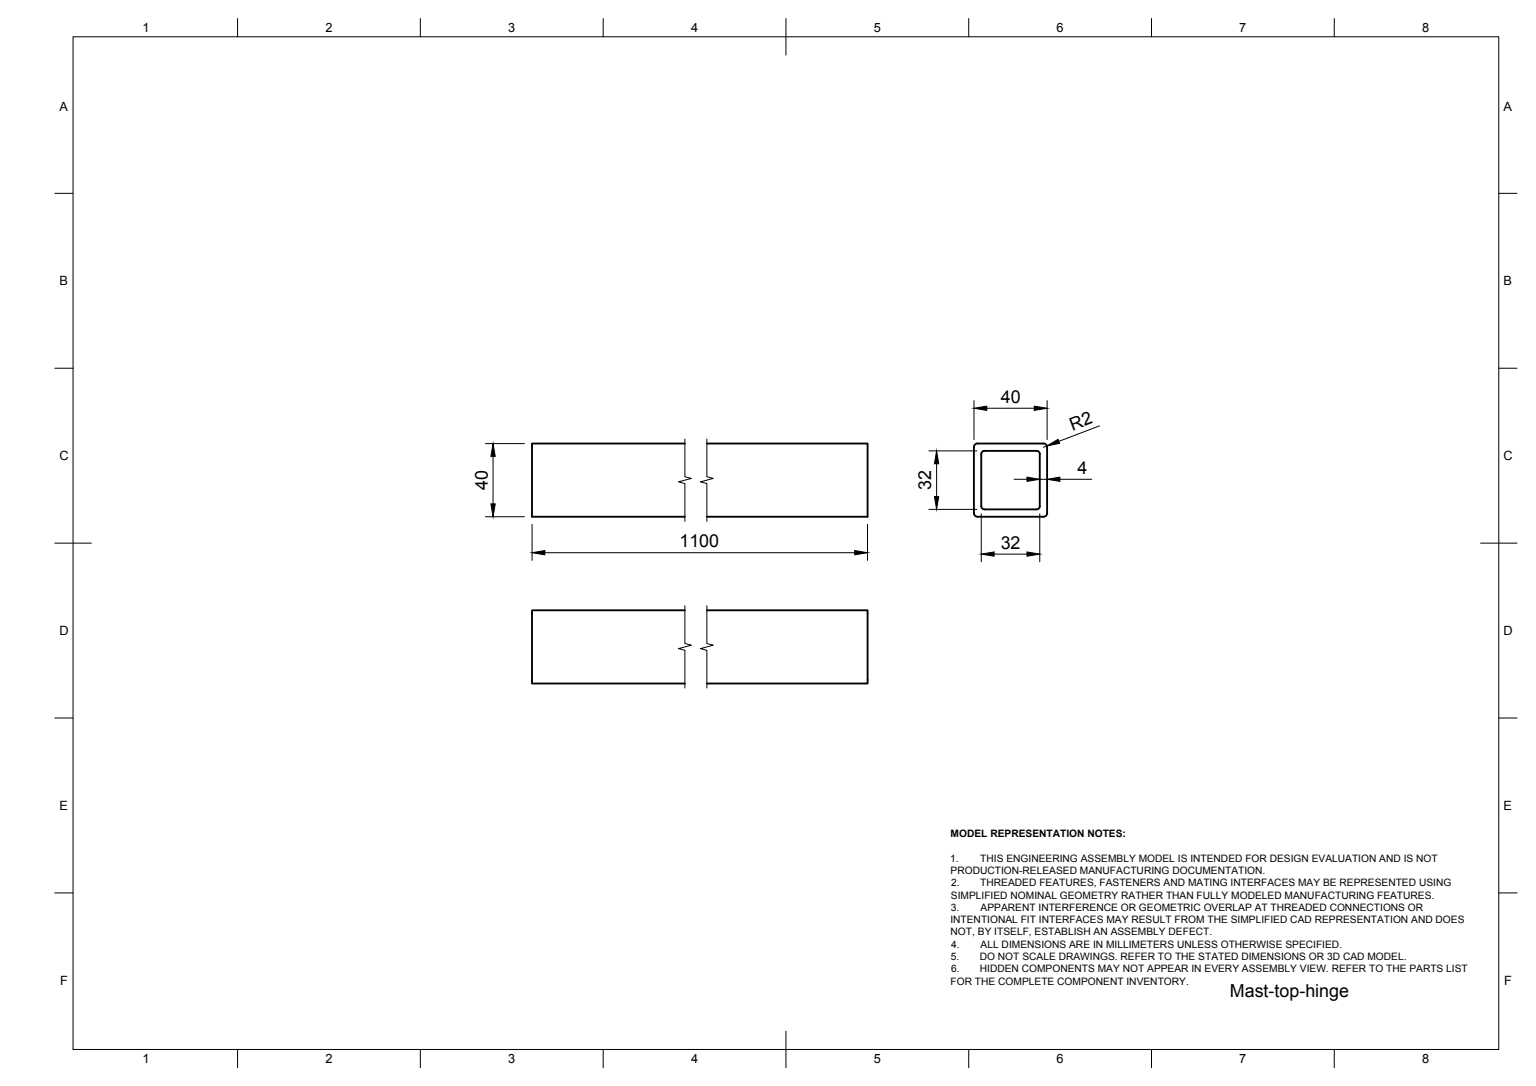
ISO-10303-21;
HEADER;
/* Generated by software containing ST-Developer
 * from STEP Tools, Inc. (www.steptools.com) 
 */

FILE_DESCRIPTION(
/* description */ (''),
/* implementation_level */ '2;1');

FILE_NAME(
/* name */ 'Mast-top-hinge.step',
/* time_stamp */ '2026-10-07T11:02:43-07:00',
/* author */ (''),
/* organization */ (''),
/* preprocessor_version */ 'ST-DEVELOPER v20.2',
/* originating_system */ 'Autodesk Translation Framework v15.15.0.0',
/* authorisation */ '');

FILE_SCHEMA (('AUTOMOTIVE_DESIGN { 1 0 10303 214 3 1 1 }'));
ENDSEC;

DATA;
#10=MECHANICAL_DESIGN_GEOMETRIC_PRESENTATION_REPRESENTATION('',(#67),#5505);
#53=SHAPE_REPRESENTATION_RELATIONSHIP('SRR','None',#5538,#60);
#60=ADVANCED_BREP_SHAPE_REPRESENTATION('',(#74),#5499);
#67=STYLED_ITEM('',(#5582),#74);
#74=MANIFOLD_SOLID_BREP('Body1',#3294);
#84=FACE_BOUND('',#447,.T.);
#85=FACE_BOUND('',#448,.T.);
#86=FACE_BOUND('',#450,.T.);
#87=FACE_BOUND('',#451,.T.);
#88=FACE_BOUND('',#461,.T.);
#89=FACE_BOUND('',#462,.T.);
#90=FACE_BOUND('',#463,.T.);
#91=FACE_BOUND('',#464,.T.);
#92=FACE_BOUND('',#466,.T.);
#93=FACE_BOUND('',#467,.T.);
#94=FACE_BOUND('',#468,.T.);
#95=FACE_BOUND('',#469,.T.);
#96=FACE_BOUND('',#477,.T.);
#97=FACE_BOUND('',#479,.T.);
#121=CYLINDRICAL_SURFACE('',#3450,2.);
#122=CYLINDRICAL_SURFACE('',#3453,2.);
#123=CYLINDRICAL_SURFACE('',#3457,2.);
#124=CYLINDRICAL_SURFACE('',#3460,2.);
#125=CYLINDRICAL_SURFACE('',#3473,1.8);
#126=CYLINDRICAL_SURFACE('',#3474,1.8);
#127=CYLINDRICAL_SURFACE('',#3476,1.8);
#128=CYLINDRICAL_SURFACE('',#3477,1.8);
#169=CIRCLE('',#3451,2.);
#170=CIRCLE('',#3452,2.);
#171=CIRCLE('',#3454,2.);
#172=CIRCLE('',#3455,2.);
#173=CIRCLE('',#3458,2.);
#174=CIRCLE('',#3459,2.);
#175=CIRCLE('',#3461,2.);
#176=CIRCLE('',#3462,2.);
#177=CIRCLE('',#3464,1.8);
#178=CIRCLE('',#3465,1.8);
#179=CIRCLE('',#3466,1.8);
#180=CIRCLE('',#3467,1.8);
#181=CIRCLE('',#3469,1.8);
#182=CIRCLE('',#3470,1.8);
#183=CIRCLE('',#3471,1.8);
#184=CIRCLE('',#3472,1.8);
#276=FACE_OUTER_BOUND('',#446,.T.);
#277=FACE_OUTER_BOUND('',#449,.T.);
#278=FACE_OUTER_BOUND('',#452,.T.);
#279=FACE_OUTER_BOUND('',#453,.T.);
#280=FACE_OUTER_BOUND('',#454,.T.);
#281=FACE_OUTER_BOUND('',#455,.T.);
#282=FACE_OUTER_BOUND('',#456,.T.);
#283=FACE_OUTER_BOUND('',#457,.T.);
#284=FACE_OUTER_BOUND('',#458,.T.);
#285=FACE_OUTER_BOUND('',#459,.T.);
#286=FACE_OUTER_BOUND('',#460,.T.);
#287=FACE_OUTER_BOUND('',#465,.T.);
#288=FACE_OUTER_BOUND('',#470,.T.);
#289=FACE_OUTER_BOUND('',#471,.T.);
#290=FACE_OUTER_BOUND('',#472,.T.);
#291=FACE_OUTER_BOUND('',#473,.T.);
#292=FACE_OUTER_BOUND('',#474,.T.);
#293=FACE_OUTER_BOUND('',#475,.T.);
#294=FACE_OUTER_BOUND('',#476,.T.);
#295=FACE_OUTER_BOUND('',#478,.T.);
#296=FACE_OUTER_BOUND('',#480,.T.);
#297=FACE_OUTER_BOUND('',#481,.T.);
#298=FACE_OUTER_BOUND('',#482,.T.);
#299=FACE_OUTER_BOUND('',#483,.T.);
#300=FACE_OUTER_BOUND('',#484,.T.);
#301=FACE_OUTER_BOUND('',#485,.T.);
#302=FACE_OUTER_BOUND('',#486,.T.);
#303=FACE_OUTER_BOUND('',#487,.T.);
#304=FACE_OUTER_BOUND('',#488,.T.);
#305=FACE_OUTER_BOUND('',#489,.T.);
#306=FACE_OUTER_BOUND('',#490,.T.);
#307=FACE_OUTER_BOUND('',#491,.T.);
#308=FACE_OUTER_BOUND('',#492,.T.);
#309=FACE_OUTER_BOUND('',#493,.T.);
#310=FACE_OUTER_BOUND('',#494,.T.);
#311=FACE_OUTER_BOUND('',#495,.T.);
#312=FACE_OUTER_BOUND('',#496,.T.);
#313=FACE_OUTER_BOUND('',#497,.T.);
#314=FACE_OUTER_BOUND('',#498,.T.);
#315=FACE_OUTER_BOUND('',#499,.T.);
#316=FACE_OUTER_BOUND('',#500,.T.);
#317=FACE_OUTER_BOUND('',#501,.T.);
#446=EDGE_LOOP('',(#2336,#2337,#2338,#2339));
#447=EDGE_LOOP('',(#2340,#2341,#2342,#2343));
#448=EDGE_LOOP('',(#2344,#2345,#2346,#2347));
#449=EDGE_LOOP('',(#2348,#2349,#2350,#2351));
#450=EDGE_LOOP('',(#2352,#2353,#2354,#2355));
#451=EDGE_LOOP('',(#2356,#2357,#2358,#2359));
#452=EDGE_LOOP('',(#2360,#2361,#2362,#2363));
#453=EDGE_LOOP('',(#2364,#2365,#2366,#2367));
#454=EDGE_LOOP('',(#2368,#2369,#2370,#2371));
#455=EDGE_LOOP('',(#2372,#2373,#2374,#2375));
#456=EDGE_LOOP('',(#2376,#2377,#2378,#2379));
#457=EDGE_LOOP('',(#2380,#2381,#2382,#2383));
#458=EDGE_LOOP('',(#2384,#2385,#2386,#2387));
#459=EDGE_LOOP('',(#2388,#2389,#2390,#2391));
#460=EDGE_LOOP('',(#2392,#2393,#2394,#2395));
#461=EDGE_LOOP('',(#2396,#2397,#2398,#2399));
#462=EDGE_LOOP('',(#2400,#2401,#2402,#2403));
#463=EDGE_LOOP('',(#2404,#2405,#2406,#2407));
#464=EDGE_LOOP('',(#2408,#2409,#2410,#2411));
#465=EDGE_LOOP('',(#2412,#2413,#2414,#2415));
#466=EDGE_LOOP('',(#2416,#2417,#2418,#2419));
#467=EDGE_LOOP('',(#2420,#2421,#2422,#2423));
#468=EDGE_LOOP('',(#2424,#2425,#2426,#2427));
#469=EDGE_LOOP('',(#2428,#2429,#2430,#2431));
#470=EDGE_LOOP('',(#2432,#2433,#2434,#2435));
#471=EDGE_LOOP('',(#2436,#2437,#2438,#2439));
#472=EDGE_LOOP('',(#2440,#2441,#2442,#2443));
#473=EDGE_LOOP('',(#2444,#2445,#2446,#2447));
#474=EDGE_LOOP('',(#2448,#2449,#2450,#2451));
#475=EDGE_LOOP('',(#2452,#2453,#2454,#2455));
#476=EDGE_LOOP('',(#2456,#2457,#2458,#2459,#2460,#2461,#2462,#2463));
#477=EDGE_LOOP('',(#2464,#2465,#2466,#2467,#2468,#2469,#2470,#2471));
#478=EDGE_LOOP('',(#2472,#2473,#2474,#2475,#2476,#2477,#2478,#2479));
#479=EDGE_LOOP('',(#2480,#2481,#2482,#2483,#2484,#2485,#2486,#2487));
#480=EDGE_LOOP('',(#2488,#2489,#2490,#2491));
#481=EDGE_LOOP('',(#2492,#2493,#2494,#2495));
#482=EDGE_LOOP('',(#2496,#2497,#2498,#2499));
#483=EDGE_LOOP('',(#2500,#2501,#2502,#2503));
#484=EDGE_LOOP('',(#2504,#2505,#2506,#2507));
#485=EDGE_LOOP('',(#2508,#2509,#2510,#2511));
#486=EDGE_LOOP('',(#2512,#2513,#2514,#2515));
#487=EDGE_LOOP('',(#2516,#2517,#2518,#2519));
#488=EDGE_LOOP('',(#2520,#2521,#2522,#2523));
#489=EDGE_LOOP('',(#2524,#2525,#2526,#2527));
#490=EDGE_LOOP('',(#2528,#2529,#2530,#2531));
#491=EDGE_LOOP('',(#2532,#2533,#2534,#2535));
#492=EDGE_LOOP('',(#2536,#2537,#2538,#2539));
#493=EDGE_LOOP('',(#2540,#2541,#2542,#2543));
#494=EDGE_LOOP('',(#2544,#2545,#2546,#2547));
#495=EDGE_LOOP('',(#2548,#2549,#2550,#2551));
#496=EDGE_LOOP('',(#2552,#2553,#2554,#2555));
#497=EDGE_LOOP('',(#2556,#2557,#2558,#2559));
#498=EDGE_LOOP('',(#2560,#2561,#2562,#2563));
#499=EDGE_LOOP('',(#2564,#2565,#2566,#2567));
#500=EDGE_LOOP('',(#2568,#2569,#2570,#2571));
#501=EDGE_LOOP('',(#2572,#2573,#2574,#2575));
#705=LINE('',#4795,#1075);
#706=LINE('',#4797,#1076);
#707=LINE('',#4799,#1077);
#708=LINE('',#4800,#1078);
#709=LINE('',#4803,#1079);
#710=LINE('',#4805,#1080);
#711=LINE('',#4807,#1081);
#712=LINE('',#4808,#1082);
#713=LINE('',#4811,#1083);
#714=LINE('',#4813,#1084);
#715=LINE('',#4815,#1085);
#716=LINE('',#4816,#1086);
#717=LINE('',#4820,#1087);
#718=LINE('',#4822,#1088);
#719=LINE('',#4824,#1089);
#720=LINE('',#4825,#1090);
#721=LINE('',#4828,#1091);
#722=LINE('',#4830,#1092);
#723=LINE('',#4832,#1093);
#724=LINE('',#4833,#1094);
#725=LINE('',#4836,#1095);
#726=LINE('',#4838,#1096);
#727=LINE('',#4840,#1097);
#728=LINE('',#4841,#1098);
#729=LINE('',#4845,#1099);
#730=LINE('',#4847,#1100);
#731=LINE('',#4849,#1101);
#732=LINE('',#4850,#1102);
#733=LINE('',#4853,#1103);
#734=LINE('',#4855,#1104);
#735=LINE('',#4856,#1105);
#736=LINE('',#4859,#1106);
#737=LINE('',#4861,#1107);
#738=LINE('',#4862,#1108);
#739=LINE('',#4864,#1109);
#740=LINE('',#4865,#1110);
#741=LINE('',#4869,#1111);
#742=LINE('',#4871,#1112);
#743=LINE('',#4873,#1113);
#744=LINE('',#4874,#1114);
#745=LINE('',#4877,#1115);
#746=LINE('',#4879,#1116);
#747=LINE('',#4880,#1117);
#748=LINE('',#4883,#1118);
#749=LINE('',#4885,#1119);
#750=LINE('',#4886,#1120);
#751=LINE('',#4888,#1121);
#752=LINE('',#4889,#1122);
#753=LINE('',#4893,#1123);
#754=LINE('',#4895,#1124);
#755=LINE('',#4897,#1125);
#756=LINE('',#4898,#1126);
#757=LINE('',#4901,#1127);
#758=LINE('',#4903,#1128);
#759=LINE('',#4905,#1129);
#760=LINE('',#4906,#1130);
#761=LINE('',#4909,#1131);
#762=LINE('',#4911,#1132);
#763=LINE('',#4913,#1133);
#764=LINE('',#4914,#1134);
#765=LINE('',#4918,#1135);
#766=LINE('',#4920,#1136);
#767=LINE('',#4922,#1137);
#768=LINE('',#4923,#1138);
#769=LINE('',#4926,#1139);
#770=LINE('',#4928,#1140);
#771=LINE('',#4930,#1141);
#772=LINE('',#4931,#1142);
#773=LINE('',#4934,#1143);
#774=LINE('',#4936,#1144);
#775=LINE('',#4938,#1145);
#776=LINE('',#4939,#1146);
#777=LINE('',#4943,#1147);
#778=LINE('',#4945,#1148);
#779=LINE('',#4947,#1149);
#780=LINE('',#4948,#1150);
#781=LINE('',#4956,#1151);
#782=LINE('',#4960,#1152);
#783=LINE('',#4962,#1153);
#784=LINE('',#4963,#1154);
#785=LINE('',#4976,#1155);
#786=LINE('',#4980,#1156);
#787=LINE('',#4985,#1157);
#788=LINE('',#4990,#1158);
#789=LINE('',#4993,#1159);
#790=LINE('',#4995,#1160);
#791=LINE('',#4997,#1161);
#792=LINE('',#5000,#1162);
#793=LINE('',#5003,#1163);
#794=LINE('',#5004,#1164);
#795=LINE('',#5006,#1165);
#796=LINE('',#5008,#1166);
#797=LINE('',#5011,#1167);
#798=LINE('',#5012,#1168);
#799=LINE('',#5014,#1169);
#800=LINE('',#5016,#1170);
#801=LINE('',#5019,#1171);
#802=LINE('',#5020,#1172);
#803=LINE('',#5022,#1173);
#804=LINE('',#5024,#1174);
#805=LINE('',#5027,#1175);
#806=LINE('',#5028,#1176);
#807=LINE('',#5030,#1177);
#808=LINE('',#5032,#1178);
#1075=VECTOR('',#3869,1000.);
#1076=VECTOR('',#3870,1000.);
#1077=VECTOR('',#3871,1000.);
#1078=VECTOR('',#3872,1000.);
#1079=VECTOR('',#3873,1000.);
#1080=VECTOR('',#3874,1000.);
#1081=VECTOR('',#3875,1000.);
#1082=VECTOR('',#3876,1000.);
#1083=VECTOR('',#3877,1000.);
#1084=VECTOR('',#3878,1000.);
#1085=VECTOR('',#3879,1000.);
#1086=VECTOR('',#3880,1000.);
#1087=VECTOR('',#3883,1000.);
#1088=VECTOR('',#3884,1000.);
#1089=VECTOR('',#3885,1000.);
#1090=VECTOR('',#3886,1000.);
#1091=VECTOR('',#3887,1000.);
#1092=VECTOR('',#3888,1000.);
#1093=VECTOR('',#3889,1000.);
#1094=VECTOR('',#3890,1000.);
#1095=VECTOR('',#3891,1000.);
#1096=VECTOR('',#3892,1000.);
#1097=VECTOR('',#3893,1000.);
#1098=VECTOR('',#3894,1000.);
#1099=VECTOR('',#3897,1000.);
#1100=VECTOR('',#3898,1000.);
#1101=VECTOR('',#3899,1000.);
#1102=VECTOR('',#3900,1000.);
#1103=VECTOR('',#3903,1000.);
#1104=VECTOR('',#3904,1000.);
#1105=VECTOR('',#3905,1000.);
#1106=VECTOR('',#3908,1000.);
#1107=VECTOR('',#3909,1000.);
#1108=VECTOR('',#3910,1000.);
#1109=VECTOR('',#3913,1000.);
#1110=VECTOR('',#3914,1000.);
#1111=VECTOR('',#3917,1000.);
#1112=VECTOR('',#3918,1000.);
#1113=VECTOR('',#3919,1000.);
#1114=VECTOR('',#3920,1000.);
#1115=VECTOR('',#3923,1000.);
#1116=VECTOR('',#3924,1000.);
#1117=VECTOR('',#3925,1000.);
#1118=VECTOR('',#3928,1000.);
#1119=VECTOR('',#3929,1000.);
#1120=VECTOR('',#3930,1000.);
#1121=VECTOR('',#3933,1000.);
#1122=VECTOR('',#3934,1000.);
#1123=VECTOR('',#3937,1000.);
#1124=VECTOR('',#3938,1000.);
#1125=VECTOR('',#3939,1000.);
#1126=VECTOR('',#3940,1000.);
#1127=VECTOR('',#3941,1000.);
#1128=VECTOR('',#3942,1000.);
#1129=VECTOR('',#3943,1000.);
#1130=VECTOR('',#3944,1000.);
#1131=VECTOR('',#3945,1000.);
#1132=VECTOR('',#3946,1000.);
#1133=VECTOR('',#3947,1000.);
#1134=VECTOR('',#3948,1000.);
#1135=VECTOR('',#3951,1000.);
#1136=VECTOR('',#3952,1000.);
#1137=VECTOR('',#3953,1000.);
#1138=VECTOR('',#3954,1000.);
#1139=VECTOR('',#3955,1000.);
#1140=VECTOR('',#3956,1000.);
#1141=VECTOR('',#3957,1000.);
#1142=VECTOR('',#3958,1000.);
#1143=VECTOR('',#3959,1000.);
#1144=VECTOR('',#3960,1000.);
#1145=VECTOR('',#3961,1000.);
#1146=VECTOR('',#3962,1000.);
#1147=VECTOR('',#3965,1000.);
#1148=VECTOR('',#3966,1000.);
#1149=VECTOR('',#3967,1000.);
#1150=VECTOR('',#3968,1000.);
#1151=VECTOR('',#3979,1000.);
#1152=VECTOR('',#3984,1000.);
#1153=VECTOR('',#3985,1000.);
#1154=VECTOR('',#3986,1000.);
#1155=VECTOR('',#4005,1000.);
#1156=VECTOR('',#4010,1000.);
#1157=VECTOR('',#4015,1000.);
#1158=VECTOR('',#4020,1000.);
#1159=VECTOR('',#4025,1000.);
#1160=VECTOR('',#4028,1000.);
#1161=VECTOR('',#4031,1000.);
#1162=VECTOR('',#4036,1000.);
#1163=VECTOR('',#4041,1000.);
#1164=VECTOR('',#4042,1000.);
#1165=VECTOR('',#4045,1000.);
#1166=VECTOR('',#4048,1000.);
#1167=VECTOR('',#4053,1000.);
#1168=VECTOR('',#4054,1000.);
#1169=VECTOR('',#4057,1000.);
#1170=VECTOR('',#4060,1000.);
#1171=VECTOR('',#4065,1000.);
#1172=VECTOR('',#4066,1000.);
#1173=VECTOR('',#4069,1000.);
#1174=VECTOR('',#4072,1000.);
#1175=VECTOR('',#4077,1000.);
#1176=VECTOR('',#4078,1000.);
#1177=VECTOR('',#4081,1000.);
#1178=VECTOR('',#4084,1000.);
#1421=VERTEX_POINT('',#4793);
#1422=VERTEX_POINT('',#4794);
#1423=VERTEX_POINT('',#4796);
#1424=VERTEX_POINT('',#4798);
#1425=VERTEX_POINT('',#4801);
#1426=VERTEX_POINT('',#4802);
#1427=VERTEX_POINT('',#4804);
#1428=VERTEX_POINT('',#4806);
#1429=VERTEX_POINT('',#4809);
#1430=VERTEX_POINT('',#4810);
#1431=VERTEX_POINT('',#4812);
#1432=VERTEX_POINT('',#4814);
#1433=VERTEX_POINT('',#4818);
#1434=VERTEX_POINT('',#4819);
#1435=VERTEX_POINT('',#4821);
#1436=VERTEX_POINT('',#4823);
#1437=VERTEX_POINT('',#4826);
#1438=VERTEX_POINT('',#4827);
#1439=VERTEX_POINT('',#4829);
#1440=VERTEX_POINT('',#4831);
#1441=VERTEX_POINT('',#4834);
#1442=VERTEX_POINT('',#4835);
#1443=VERTEX_POINT('',#4837);
#1444=VERTEX_POINT('',#4839);
#1445=VERTEX_POINT('',#4843);
#1446=VERTEX_POINT('',#4844);
#1447=VERTEX_POINT('',#4846);
#1448=VERTEX_POINT('',#4848);
#1449=VERTEX_POINT('',#4852);
#1450=VERTEX_POINT('',#4854);
#1451=VERTEX_POINT('',#4858);
#1452=VERTEX_POINT('',#4860);
#1453=VERTEX_POINT('',#4867);
#1454=VERTEX_POINT('',#4868);
#1455=VERTEX_POINT('',#4870);
#1456=VERTEX_POINT('',#4872);
#1457=VERTEX_POINT('',#4876);
#1458=VERTEX_POINT('',#4878);
#1459=VERTEX_POINT('',#4882);
#1460=VERTEX_POINT('',#4884);
#1461=VERTEX_POINT('',#4891);
#1462=VERTEX_POINT('',#4892);
#1463=VERTEX_POINT('',#4894);
#1464=VERTEX_POINT('',#4896);
#1465=VERTEX_POINT('',#4899);
#1466=VERTEX_POINT('',#4900);
#1467=VERTEX_POINT('',#4902);
#1468=VERTEX_POINT('',#4904);
#1469=VERTEX_POINT('',#4907);
#1470=VERTEX_POINT('',#4908);
#1471=VERTEX_POINT('',#4910);
#1472=VERTEX_POINT('',#4912);
#1473=VERTEX_POINT('',#4916);
#1474=VERTEX_POINT('',#4917);
#1475=VERTEX_POINT('',#4919);
#1476=VERTEX_POINT('',#4921);
#1477=VERTEX_POINT('',#4924);
#1478=VERTEX_POINT('',#4925);
#1479=VERTEX_POINT('',#4927);
#1480=VERTEX_POINT('',#4929);
#1481=VERTEX_POINT('',#4932);
#1482=VERTEX_POINT('',#4933);
#1483=VERTEX_POINT('',#4935);
#1484=VERTEX_POINT('',#4937);
#1485=VERTEX_POINT('',#4941);
#1486=VERTEX_POINT('',#4942);
#1487=VERTEX_POINT('',#4944);
#1488=VERTEX_POINT('',#4946);
#1489=VERTEX_POINT('',#4953);
#1490=VERTEX_POINT('',#4955);
#1491=VERTEX_POINT('',#4959);
#1492=VERTEX_POINT('',#4961);
#1493=VERTEX_POINT('',#4971);
#1494=VERTEX_POINT('',#4973);
#1495=VERTEX_POINT('',#4975);
#1496=VERTEX_POINT('',#4978);
#1497=VERTEX_POINT('',#4982);
#1498=VERTEX_POINT('',#4984);
#1499=VERTEX_POINT('',#4987);
#1500=VERTEX_POINT('',#4989);
#1763=EDGE_CURVE('',#1421,#1422,#705,.T.);
#1764=EDGE_CURVE('',#1422,#1423,#706,.T.);
#1765=EDGE_CURVE('',#1424,#1423,#707,.T.);
#1766=EDGE_CURVE('',#1421,#1424,#708,.T.);
#1767=EDGE_CURVE('',#1425,#1426,#709,.T.);
#1768=EDGE_CURVE('',#1425,#1427,#710,.T.);
#1769=EDGE_CURVE('',#1427,#1428,#711,.T.);
#1770=EDGE_CURVE('',#1426,#1428,#712,.T.);
#1771=EDGE_CURVE('',#1429,#1430,#713,.T.);
#1772=EDGE_CURVE('',#1430,#1431,#714,.T.);
#1773=EDGE_CURVE('',#1432,#1431,#715,.T.);
#1774=EDGE_CURVE('',#1429,#1432,#716,.T.);
#1775=EDGE_CURVE('',#1433,#1434,#717,.T.);
#1776=EDGE_CURVE('',#1435,#1434,#718,.T.);
#1777=EDGE_CURVE('',#1436,#1435,#719,.T.);
#1778=EDGE_CURVE('',#1436,#1433,#720,.T.);
#1779=EDGE_CURVE('',#1437,#1438,#721,.T.);
#1780=EDGE_CURVE('',#1438,#1439,#722,.T.);
#1781=EDGE_CURVE('',#1440,#1439,#723,.T.);
#1782=EDGE_CURVE('',#1437,#1440,#724,.T.);
#1783=EDGE_CURVE('',#1441,#1442,#725,.T.);
#1784=EDGE_CURVE('',#1441,#1443,#726,.T.);
#1785=EDGE_CURVE('',#1443,#1444,#727,.T.);
#1786=EDGE_CURVE('',#1442,#1444,#728,.T.);
#1787=EDGE_CURVE('',#1445,#1446,#729,.T.);
#1788=EDGE_CURVE('',#1445,#1447,#730,.T.);
#1789=EDGE_CURVE('',#1447,#1448,#731,.T.);
#1790=EDGE_CURVE('',#1448,#1446,#732,.T.);
#1791=EDGE_CURVE('',#1447,#1449,#733,.T.);
#1792=EDGE_CURVE('',#1449,#1450,#734,.T.);
#1793=EDGE_CURVE('',#1450,#1448,#735,.T.);
#1794=EDGE_CURVE('',#1449,#1451,#736,.T.);
#1795=EDGE_CURVE('',#1451,#1452,#737,.T.);
#1796=EDGE_CURVE('',#1452,#1450,#738,.T.);
#1797=EDGE_CURVE('',#1451,#1445,#739,.T.);
#1798=EDGE_CURVE('',#1446,#1452,#740,.T.);
#1799=EDGE_CURVE('',#1453,#1454,#741,.T.);
#1800=EDGE_CURVE('',#1453,#1455,#742,.T.);
#1801=EDGE_CURVE('',#1455,#1456,#743,.T.);
#1802=EDGE_CURVE('',#1456,#1454,#744,.T.);
#1803=EDGE_CURVE('',#1457,#1455,#745,.T.);
#1804=EDGE_CURVE('',#1457,#1458,#746,.T.);
#1805=EDGE_CURVE('',#1456,#1458,#747,.T.);
#1806=EDGE_CURVE('',#1459,#1457,#748,.T.);
#1807=EDGE_CURVE('',#1459,#1460,#749,.T.);
#1808=EDGE_CURVE('',#1458,#1460,#750,.T.);
#1809=EDGE_CURVE('',#1459,#1453,#751,.T.);
#1810=EDGE_CURVE('',#1454,#1460,#752,.T.);
#1811=EDGE_CURVE('',#1461,#1462,#753,.T.);
#1812=EDGE_CURVE('',#1463,#1462,#754,.T.);
#1813=EDGE_CURVE('',#1464,#1463,#755,.T.);
#1814=EDGE_CURVE('',#1464,#1461,#756,.T.);
#1815=EDGE_CURVE('',#1465,#1466,#757,.T.);
#1816=EDGE_CURVE('',#1466,#1467,#758,.T.);
#1817=EDGE_CURVE('',#1467,#1468,#759,.T.);
#1818=EDGE_CURVE('',#1468,#1465,#760,.T.);
#1819=EDGE_CURVE('',#1469,#1470,#761,.T.);
#1820=EDGE_CURVE('',#1469,#1471,#762,.T.);
#1821=EDGE_CURVE('',#1471,#1472,#763,.T.);
#1822=EDGE_CURVE('',#1470,#1472,#764,.T.);
#1823=EDGE_CURVE('',#1473,#1474,#765,.T.);
#1824=EDGE_CURVE('',#1475,#1474,#766,.F.);
#1825=EDGE_CURVE('',#1476,#1475,#767,.T.);
#1826=EDGE_CURVE('',#1476,#1473,#768,.F.);
#1827=EDGE_CURVE('',#1477,#1478,#769,.T.);
#1828=EDGE_CURVE('',#1478,#1479,#770,.T.);
#1829=EDGE_CURVE('',#1479,#1480,#771,.T.);
#1830=EDGE_CURVE('',#1480,#1477,#772,.T.);
#1831=EDGE_CURVE('',#1481,#1482,#773,.T.);
#1832=EDGE_CURVE('',#1482,#1483,#774,.T.);
#1833=EDGE_CURVE('',#1484,#1483,#775,.T.);
#1834=EDGE_CURVE('',#1481,#1484,#776,.T.);
#1835=EDGE_CURVE('',#1485,#1486,#777,.T.);
#1836=EDGE_CURVE('',#1487,#1485,#778,.T.);
#1837=EDGE_CURVE('',#1487,#1488,#779,.T.);
#1838=EDGE_CURVE('',#1488,#1486,#780,.T.);
#1839=EDGE_CURVE('',#1474,#1485,#169,.T.);
#1840=EDGE_CURVE('',#1473,#1487,#170,.T.);
#1841=EDGE_CURVE('',#1489,#1475,#171,.T.);
#1842=EDGE_CURVE('',#1490,#1489,#781,.T.);
#1843=EDGE_CURVE('',#1490,#1476,#172,.T.);
#1844=EDGE_CURVE('',#1491,#1489,#782,.F.);
#1845=EDGE_CURVE('',#1492,#1491,#783,.T.);
#1846=EDGE_CURVE('',#1492,#1490,#784,.F.);
#1847=EDGE_CURVE('',#1434,#1491,#173,.T.);
#1848=EDGE_CURVE('',#1433,#1492,#174,.T.);
#1849=EDGE_CURVE('',#1486,#1435,#175,.T.);
#1850=EDGE_CURVE('',#1488,#1436,#176,.T.);
#1851=EDGE_CURVE('',#1423,#1493,#177,.T.);
#1852=EDGE_CURVE('',#1494,#1422,#178,.T.);
#1853=EDGE_CURVE('',#1495,#1494,#785,.T.);
#1854=EDGE_CURVE('',#1463,#1495,#179,.T.);
#1855=EDGE_CURVE('',#1496,#1462,#180,.T.);
#1856=EDGE_CURVE('',#1496,#1493,#786,.T.);
#1857=EDGE_CURVE('',#1424,#1497,#181,.T.);
#1858=EDGE_CURVE('',#1498,#1497,#787,.T.);
#1859=EDGE_CURVE('',#1498,#1461,#182,.T.);
#1860=EDGE_CURVE('',#1464,#1499,#183,.T.);
#1861=EDGE_CURVE('',#1499,#1500,#788,.T.);
#1862=EDGE_CURVE('',#1500,#1421,#184,.T.);
#1863=EDGE_CURVE('',#1498,#1496,#789,.T.);
#1864=EDGE_CURVE('',#1499,#1495,#790,.T.);
#1865=EDGE_CURVE('',#1500,#1494,#791,.T.);
#1866=EDGE_CURVE('',#1497,#1493,#792,.T.);
#1867=EDGE_CURVE('',#1466,#1479,#793,.T.);
#1868=EDGE_CURVE('',#1467,#1478,#794,.T.);
#1869=EDGE_CURVE('',#1468,#1477,#795,.T.);
#1870=EDGE_CURVE('',#1465,#1480,#796,.T.);
#1871=EDGE_CURVE('',#1469,#1483,#797,.T.);
#1872=EDGE_CURVE('',#1471,#1482,#798,.T.);
#1873=EDGE_CURVE('',#1472,#1481,#799,.T.);
#1874=EDGE_CURVE('',#1470,#1484,#800,.T.);
#1875=EDGE_CURVE('',#1425,#1439,#801,.T.);
#1876=EDGE_CURVE('',#1427,#1438,#802,.T.);
#1877=EDGE_CURVE('',#1428,#1437,#803,.T.);
#1878=EDGE_CURVE('',#1426,#1440,#804,.T.);
#1879=EDGE_CURVE('',#1430,#1443,#805,.T.);
#1880=EDGE_CURVE('',#1431,#1441,#806,.T.);
#1881=EDGE_CURVE('',#1432,#1442,#807,.T.);
#1882=EDGE_CURVE('',#1429,#1444,#808,.T.);
#2336=ORIENTED_EDGE('',*,*,#1763,.T.);
#2337=ORIENTED_EDGE('',*,*,#1764,.T.);
#2338=ORIENTED_EDGE('',*,*,#1765,.F.);
#2339=ORIENTED_EDGE('',*,*,#1766,.F.);
#2340=ORIENTED_EDGE('',*,*,#1767,.F.);
#2341=ORIENTED_EDGE('',*,*,#1768,.T.);
#2342=ORIENTED_EDGE('',*,*,#1769,.T.);
#2343=ORIENTED_EDGE('',*,*,#1770,.F.);
#2344=ORIENTED_EDGE('',*,*,#1771,.T.);
#2345=ORIENTED_EDGE('',*,*,#1772,.T.);
#2346=ORIENTED_EDGE('',*,*,#1773,.F.);
#2347=ORIENTED_EDGE('',*,*,#1774,.F.);
#2348=ORIENTED_EDGE('',*,*,#1775,.T.);
#2349=ORIENTED_EDGE('',*,*,#1776,.F.);
#2350=ORIENTED_EDGE('',*,*,#1777,.F.);
#2351=ORIENTED_EDGE('',*,*,#1778,.T.);
#2352=ORIENTED_EDGE('',*,*,#1779,.T.);
#2353=ORIENTED_EDGE('',*,*,#1780,.T.);
#2354=ORIENTED_EDGE('',*,*,#1781,.F.);
#2355=ORIENTED_EDGE('',*,*,#1782,.F.);
#2356=ORIENTED_EDGE('',*,*,#1783,.F.);
#2357=ORIENTED_EDGE('',*,*,#1784,.T.);
#2358=ORIENTED_EDGE('',*,*,#1785,.T.);
#2359=ORIENTED_EDGE('',*,*,#1786,.F.);
#2360=ORIENTED_EDGE('',*,*,#1787,.F.);
#2361=ORIENTED_EDGE('',*,*,#1788,.T.);
#2362=ORIENTED_EDGE('',*,*,#1789,.T.);
#2363=ORIENTED_EDGE('',*,*,#1790,.T.);
#2364=ORIENTED_EDGE('',*,*,#1789,.F.);
#2365=ORIENTED_EDGE('',*,*,#1791,.T.);
#2366=ORIENTED_EDGE('',*,*,#1792,.T.);
#2367=ORIENTED_EDGE('',*,*,#1793,.T.);
#2368=ORIENTED_EDGE('',*,*,#1792,.F.);
#2369=ORIENTED_EDGE('',*,*,#1794,.T.);
#2370=ORIENTED_EDGE('',*,*,#1795,.T.);
#2371=ORIENTED_EDGE('',*,*,#1796,.T.);
#2372=ORIENTED_EDGE('',*,*,#1795,.F.);
#2373=ORIENTED_EDGE('',*,*,#1797,.T.);
#2374=ORIENTED_EDGE('',*,*,#1787,.T.);
#2375=ORIENTED_EDGE('',*,*,#1798,.T.);
#2376=ORIENTED_EDGE('',*,*,#1799,.F.);
#2377=ORIENTED_EDGE('',*,*,#1800,.T.);
#2378=ORIENTED_EDGE('',*,*,#1801,.T.);
#2379=ORIENTED_EDGE('',*,*,#1802,.T.);
#2380=ORIENTED_EDGE('',*,*,#1803,.F.);
#2381=ORIENTED_EDGE('',*,*,#1804,.T.);
#2382=ORIENTED_EDGE('',*,*,#1805,.F.);
#2383=ORIENTED_EDGE('',*,*,#1801,.F.);
#2384=ORIENTED_EDGE('',*,*,#1806,.F.);
#2385=ORIENTED_EDGE('',*,*,#1807,.T.);
#2386=ORIENTED_EDGE('',*,*,#1808,.F.);
#2387=ORIENTED_EDGE('',*,*,#1804,.F.);
#2388=ORIENTED_EDGE('',*,*,#1807,.F.);
#2389=ORIENTED_EDGE('',*,*,#1809,.T.);
#2390=ORIENTED_EDGE('',*,*,#1799,.T.);
#2391=ORIENTED_EDGE('',*,*,#1810,.T.);
#2392=ORIENTED_EDGE('',*,*,#1811,.T.);
#2393=ORIENTED_EDGE('',*,*,#1812,.F.);
#2394=ORIENTED_EDGE('',*,*,#1813,.F.);
#2395=ORIENTED_EDGE('',*,*,#1814,.T.);
#2396=ORIENTED_EDGE('',*,*,#1815,.T.);
#2397=ORIENTED_EDGE('',*,*,#1816,.T.);
#2398=ORIENTED_EDGE('',*,*,#1817,.T.);
#2399=ORIENTED_EDGE('',*,*,#1818,.T.);
#2400=ORIENTED_EDGE('',*,*,#1819,.F.);
#2401=ORIENTED_EDGE('',*,*,#1820,.T.);
#2402=ORIENTED_EDGE('',*,*,#1821,.T.);
#2403=ORIENTED_EDGE('',*,*,#1822,.F.);
#2404=ORIENTED_EDGE('',*,*,#1806,.T.);
#2405=ORIENTED_EDGE('',*,*,#1803,.T.);
#2406=ORIENTED_EDGE('',*,*,#1800,.F.);
#2407=ORIENTED_EDGE('',*,*,#1809,.F.);
#2408=ORIENTED_EDGE('',*,*,#1794,.F.);
#2409=ORIENTED_EDGE('',*,*,#1791,.F.);
#2410=ORIENTED_EDGE('',*,*,#1788,.F.);
#2411=ORIENTED_EDGE('',*,*,#1797,.F.);
#2412=ORIENTED_EDGE('',*,*,#1823,.T.);
#2413=ORIENTED_EDGE('',*,*,#1824,.F.);
#2414=ORIENTED_EDGE('',*,*,#1825,.F.);
#2415=ORIENTED_EDGE('',*,*,#1826,.T.);
#2416=ORIENTED_EDGE('',*,*,#1827,.T.);
#2417=ORIENTED_EDGE('',*,*,#1828,.T.);
#2418=ORIENTED_EDGE('',*,*,#1829,.T.);
#2419=ORIENTED_EDGE('',*,*,#1830,.T.);
#2420=ORIENTED_EDGE('',*,*,#1831,.T.);
#2421=ORIENTED_EDGE('',*,*,#1832,.T.);
#2422=ORIENTED_EDGE('',*,*,#1833,.F.);
#2423=ORIENTED_EDGE('',*,*,#1834,.F.);
#2424=ORIENTED_EDGE('',*,*,#1802,.F.);
#2425=ORIENTED_EDGE('',*,*,#1805,.T.);
#2426=ORIENTED_EDGE('',*,*,#1808,.T.);
#2427=ORIENTED_EDGE('',*,*,#1810,.F.);
#2428=ORIENTED_EDGE('',*,*,#1790,.F.);
#2429=ORIENTED_EDGE('',*,*,#1793,.F.);
#2430=ORIENTED_EDGE('',*,*,#1796,.F.);
#2431=ORIENTED_EDGE('',*,*,#1798,.F.);
#2432=ORIENTED_EDGE('',*,*,#1835,.F.);
#2433=ORIENTED_EDGE('',*,*,#1836,.F.);
#2434=ORIENTED_EDGE('',*,*,#1837,.T.);
#2435=ORIENTED_EDGE('',*,*,#1838,.T.);
#2436=ORIENTED_EDGE('',*,*,#1836,.T.);
#2437=ORIENTED_EDGE('',*,*,#1839,.F.);
#2438=ORIENTED_EDGE('',*,*,#1823,.F.);
#2439=ORIENTED_EDGE('',*,*,#1840,.T.);
#2440=ORIENTED_EDGE('',*,*,#1825,.T.);
#2441=ORIENTED_EDGE('',*,*,#1841,.F.);
#2442=ORIENTED_EDGE('',*,*,#1842,.F.);
#2443=ORIENTED_EDGE('',*,*,#1843,.T.);
#2444=ORIENTED_EDGE('',*,*,#1842,.T.);
#2445=ORIENTED_EDGE('',*,*,#1844,.F.);
#2446=ORIENTED_EDGE('',*,*,#1845,.F.);
#2447=ORIENTED_EDGE('',*,*,#1846,.T.);
#2448=ORIENTED_EDGE('',*,*,#1845,.T.);
#2449=ORIENTED_EDGE('',*,*,#1847,.F.);
#2450=ORIENTED_EDGE('',*,*,#1775,.F.);
#2451=ORIENTED_EDGE('',*,*,#1848,.T.);
#2452=ORIENTED_EDGE('',*,*,#1777,.T.);
#2453=ORIENTED_EDGE('',*,*,#1849,.F.);
#2454=ORIENTED_EDGE('',*,*,#1838,.F.);
#2455=ORIENTED_EDGE('',*,*,#1850,.T.);
#2456=ORIENTED_EDGE('',*,*,#1776,.T.);
#2457=ORIENTED_EDGE('',*,*,#1847,.T.);
#2458=ORIENTED_EDGE('',*,*,#1844,.T.);
#2459=ORIENTED_EDGE('',*,*,#1841,.T.);
#2460=ORIENTED_EDGE('',*,*,#1824,.T.);
#2461=ORIENTED_EDGE('',*,*,#1839,.T.);
#2462=ORIENTED_EDGE('',*,*,#1835,.T.);
#2463=ORIENTED_EDGE('',*,*,#1849,.T.);
#2464=ORIENTED_EDGE('',*,*,#1851,.F.);
#2465=ORIENTED_EDGE('',*,*,#1764,.F.);
#2466=ORIENTED_EDGE('',*,*,#1852,.F.);
#2467=ORIENTED_EDGE('',*,*,#1853,.F.);
#2468=ORIENTED_EDGE('',*,*,#1854,.F.);
#2469=ORIENTED_EDGE('',*,*,#1812,.T.);
#2470=ORIENTED_EDGE('',*,*,#1855,.F.);
#2471=ORIENTED_EDGE('',*,*,#1856,.T.);
#2472=ORIENTED_EDGE('',*,*,#1778,.F.);
#2473=ORIENTED_EDGE('',*,*,#1850,.F.);
#2474=ORIENTED_EDGE('',*,*,#1837,.F.);
#2475=ORIENTED_EDGE('',*,*,#1840,.F.);
#2476=ORIENTED_EDGE('',*,*,#1826,.F.);
#2477=ORIENTED_EDGE('',*,*,#1843,.F.);
#2478=ORIENTED_EDGE('',*,*,#1846,.F.);
#2479=ORIENTED_EDGE('',*,*,#1848,.F.);
#2480=ORIENTED_EDGE('',*,*,#1857,.T.);
#2481=ORIENTED_EDGE('',*,*,#1858,.F.);
#2482=ORIENTED_EDGE('',*,*,#1859,.T.);
#2483=ORIENTED_EDGE('',*,*,#1814,.F.);
#2484=ORIENTED_EDGE('',*,*,#1860,.T.);
#2485=ORIENTED_EDGE('',*,*,#1861,.T.);
#2486=ORIENTED_EDGE('',*,*,#1862,.T.);
#2487=ORIENTED_EDGE('',*,*,#1766,.T.);
#2488=ORIENTED_EDGE('',*,*,#1855,.T.);
#2489=ORIENTED_EDGE('',*,*,#1811,.F.);
#2490=ORIENTED_EDGE('',*,*,#1859,.F.);
#2491=ORIENTED_EDGE('',*,*,#1863,.T.);
#2492=ORIENTED_EDGE('',*,*,#1813,.T.);
#2493=ORIENTED_EDGE('',*,*,#1854,.T.);
#2494=ORIENTED_EDGE('',*,*,#1864,.F.);
#2495=ORIENTED_EDGE('',*,*,#1860,.F.);
#2496=ORIENTED_EDGE('',*,*,#1864,.T.);
#2497=ORIENTED_EDGE('',*,*,#1853,.T.);
#2498=ORIENTED_EDGE('',*,*,#1865,.F.);
#2499=ORIENTED_EDGE('',*,*,#1861,.F.);
#2500=ORIENTED_EDGE('',*,*,#1865,.T.);
#2501=ORIENTED_EDGE('',*,*,#1852,.T.);
#2502=ORIENTED_EDGE('',*,*,#1763,.F.);
#2503=ORIENTED_EDGE('',*,*,#1862,.F.);
#2504=ORIENTED_EDGE('',*,*,#1765,.T.);
#2505=ORIENTED_EDGE('',*,*,#1851,.T.);
#2506=ORIENTED_EDGE('',*,*,#1866,.F.);
#2507=ORIENTED_EDGE('',*,*,#1857,.F.);
#2508=ORIENTED_EDGE('',*,*,#1866,.T.);
#2509=ORIENTED_EDGE('',*,*,#1856,.F.);
#2510=ORIENTED_EDGE('',*,*,#1863,.F.);
#2511=ORIENTED_EDGE('',*,*,#1858,.T.);
#2512=ORIENTED_EDGE('',*,*,#1867,.T.);
#2513=ORIENTED_EDGE('',*,*,#1828,.F.);
#2514=ORIENTED_EDGE('',*,*,#1868,.F.);
#2515=ORIENTED_EDGE('',*,*,#1816,.F.);
#2516=ORIENTED_EDGE('',*,*,#1868,.T.);
#2517=ORIENTED_EDGE('',*,*,#1827,.F.);
#2518=ORIENTED_EDGE('',*,*,#1869,.F.);
#2519=ORIENTED_EDGE('',*,*,#1817,.F.);
#2520=ORIENTED_EDGE('',*,*,#1869,.T.);
#2521=ORIENTED_EDGE('',*,*,#1830,.F.);
#2522=ORIENTED_EDGE('',*,*,#1870,.F.);
#2523=ORIENTED_EDGE('',*,*,#1818,.F.);
#2524=ORIENTED_EDGE('',*,*,#1870,.T.);
#2525=ORIENTED_EDGE('',*,*,#1829,.F.);
#2526=ORIENTED_EDGE('',*,*,#1867,.F.);
#2527=ORIENTED_EDGE('',*,*,#1815,.F.);
#2528=ORIENTED_EDGE('',*,*,#1871,.T.);
#2529=ORIENTED_EDGE('',*,*,#1832,.F.);
#2530=ORIENTED_EDGE('',*,*,#1872,.F.);
#2531=ORIENTED_EDGE('',*,*,#1820,.F.);
#2532=ORIENTED_EDGE('',*,*,#1872,.T.);
#2533=ORIENTED_EDGE('',*,*,#1831,.F.);
#2534=ORIENTED_EDGE('',*,*,#1873,.F.);
#2535=ORIENTED_EDGE('',*,*,#1821,.F.);
#2536=ORIENTED_EDGE('',*,*,#1822,.T.);
#2537=ORIENTED_EDGE('',*,*,#1873,.T.);
#2538=ORIENTED_EDGE('',*,*,#1834,.T.);
#2539=ORIENTED_EDGE('',*,*,#1874,.F.);
#2540=ORIENTED_EDGE('',*,*,#1819,.T.);
#2541=ORIENTED_EDGE('',*,*,#1874,.T.);
#2542=ORIENTED_EDGE('',*,*,#1833,.T.);
#2543=ORIENTED_EDGE('',*,*,#1871,.F.);
#2544=ORIENTED_EDGE('',*,*,#1875,.T.);
#2545=ORIENTED_EDGE('',*,*,#1780,.F.);
#2546=ORIENTED_EDGE('',*,*,#1876,.F.);
#2547=ORIENTED_EDGE('',*,*,#1768,.F.);
#2548=ORIENTED_EDGE('',*,*,#1876,.T.);
#2549=ORIENTED_EDGE('',*,*,#1779,.F.);
#2550=ORIENTED_EDGE('',*,*,#1877,.F.);
#2551=ORIENTED_EDGE('',*,*,#1769,.F.);
#2552=ORIENTED_EDGE('',*,*,#1770,.T.);
#2553=ORIENTED_EDGE('',*,*,#1877,.T.);
#2554=ORIENTED_EDGE('',*,*,#1782,.T.);
#2555=ORIENTED_EDGE('',*,*,#1878,.F.);
#2556=ORIENTED_EDGE('',*,*,#1767,.T.);
#2557=ORIENTED_EDGE('',*,*,#1878,.T.);
#2558=ORIENTED_EDGE('',*,*,#1781,.T.);
#2559=ORIENTED_EDGE('',*,*,#1875,.F.);
#2560=ORIENTED_EDGE('',*,*,#1879,.T.);
#2561=ORIENTED_EDGE('',*,*,#1784,.F.);
#2562=ORIENTED_EDGE('',*,*,#1880,.F.);
#2563=ORIENTED_EDGE('',*,*,#1772,.F.);
#2564=ORIENTED_EDGE('',*,*,#1773,.T.);
#2565=ORIENTED_EDGE('',*,*,#1880,.T.);
#2566=ORIENTED_EDGE('',*,*,#1783,.T.);
#2567=ORIENTED_EDGE('',*,*,#1881,.F.);
#2568=ORIENTED_EDGE('',*,*,#1774,.T.);
#2569=ORIENTED_EDGE('',*,*,#1881,.T.);
#2570=ORIENTED_EDGE('',*,*,#1786,.T.);
#2571=ORIENTED_EDGE('',*,*,#1882,.F.);
#2572=ORIENTED_EDGE('',*,*,#1882,.T.);
#2573=ORIENTED_EDGE('',*,*,#1785,.F.);
#2574=ORIENTED_EDGE('',*,*,#1879,.F.);
#2575=ORIENTED_EDGE('',*,*,#1771,.F.);
#3034=PLANE('',#3437);
#3035=PLANE('',#3438);
#3036=PLANE('',#3439);
#3037=PLANE('',#3440);
#3038=PLANE('',#3441);
#3039=PLANE('',#3442);
#3040=PLANE('',#3443);
#3041=PLANE('',#3444);
#3042=PLANE('',#3445);
#3043=PLANE('',#3446);
#3044=PLANE('',#3447);
#3045=PLANE('',#3448);
#3046=PLANE('',#3449);
#3047=PLANE('',#3456);
#3048=PLANE('',#3463);
#3049=PLANE('',#3468);
#3050=PLANE('',#3475);
#3051=PLANE('',#3478);
#3052=PLANE('',#3479);
#3053=PLANE('',#3480);
#3054=PLANE('',#3481);
#3055=PLANE('',#3482);
#3056=PLANE('',#3483);
#3057=PLANE('',#3484);
#3058=PLANE('',#3485);
#3059=PLANE('',#3486);
#3060=PLANE('',#3487);
#3061=PLANE('',#3488);
#3062=PLANE('',#3489);
#3063=PLANE('',#3490);
#3064=PLANE('',#3491);
#3065=PLANE('',#3492);
#3066=PLANE('',#3493);
#3067=PLANE('',#3494);
#3167=ADVANCED_FACE('',(#276,#84,#85),#3034,.T.);
#3168=ADVANCED_FACE('',(#277,#86,#87),#3035,.T.);
#3169=ADVANCED_FACE('',(#278),#3036,.T.);
#3170=ADVANCED_FACE('',(#279),#3037,.T.);
#3171=ADVANCED_FACE('',(#280),#3038,.T.);
#3172=ADVANCED_FACE('',(#281),#3039,.T.);
#3173=ADVANCED_FACE('',(#282),#3040,.T.);
#3174=ADVANCED_FACE('',(#283),#3041,.F.);
#3175=ADVANCED_FACE('',(#284),#3042,.F.);
#3176=ADVANCED_FACE('',(#285),#3043,.T.);
#3177=ADVANCED_FACE('',(#286,#88,#89,#90,#91),#3044,.T.);
#3178=ADVANCED_FACE('',(#287,#92,#93,#94,#95),#3045,.T.);
#3179=ADVANCED_FACE('',(#288),#3046,.T.);
#3180=ADVANCED_FACE('',(#289),#121,.T.);
#3181=ADVANCED_FACE('',(#290),#122,.T.);
#3182=ADVANCED_FACE('',(#291),#3047,.T.);
#3183=ADVANCED_FACE('',(#292),#123,.T.);
#3184=ADVANCED_FACE('',(#293),#124,.T.);
#3185=ADVANCED_FACE('',(#294,#96),#3048,.T.);
#3186=ADVANCED_FACE('',(#295,#97),#3049,.F.);
#3187=ADVANCED_FACE('',(#296),#125,.F.);
#3188=ADVANCED_FACE('',(#297),#126,.F.);
#3189=ADVANCED_FACE('',(#298),#3050,.T.);
#3190=ADVANCED_FACE('',(#299),#127,.F.);
#3191=ADVANCED_FACE('',(#300),#128,.F.);
#3192=ADVANCED_FACE('',(#301),#3051,.T.);
#3193=ADVANCED_FACE('',(#302),#3052,.T.);
#3194=ADVANCED_FACE('',(#303),#3053,.T.);
#3195=ADVANCED_FACE('',(#304),#3054,.T.);
#3196=ADVANCED_FACE('',(#305),#3055,.T.);
#3197=ADVANCED_FACE('',(#306),#3056,.T.);
#3198=ADVANCED_FACE('',(#307),#3057,.T.);
#3199=ADVANCED_FACE('',(#308),#3058,.F.);
#3200=ADVANCED_FACE('',(#309),#3059,.F.);
#3201=ADVANCED_FACE('',(#310),#3060,.T.);
#3202=ADVANCED_FACE('',(#311),#3061,.T.);
#3203=ADVANCED_FACE('',(#312),#3062,.F.);
#3204=ADVANCED_FACE('',(#313),#3063,.F.);
#3205=ADVANCED_FACE('',(#314),#3064,.T.);
#3206=ADVANCED_FACE('',(#315),#3065,.F.);
#3207=ADVANCED_FACE('',(#316),#3066,.F.);
#3208=ADVANCED_FACE('',(#317),#3067,.T.);
#3294=CLOSED_SHELL('',(#3167,#3168,#3169,#3170,#3171,#3172,#3173,#3174,
#3175,#3176,#3177,#3178,#3179,#3180,#3181,#3182,#3183,#3184,#3185,#3186,
#3187,#3188,#3189,#3190,#3191,#3192,#3193,#3194,#3195,#3196,#3197,#3198,
#3199,#3200,#3201,#3202,#3203,#3204,#3205,#3206,#3207,#3208));
#3436=AXIS2_PLACEMENT_3D('',#4791,#3865,#3866);
#3437=AXIS2_PLACEMENT_3D('',#4792,#3867,#3868);
#3438=AXIS2_PLACEMENT_3D('',#4817,#3881,#3882);
#3439=AXIS2_PLACEMENT_3D('',#4842,#3895,#3896);
#3440=AXIS2_PLACEMENT_3D('',#4851,#3901,#3902);
#3441=AXIS2_PLACEMENT_3D('',#4857,#3906,#3907);
#3442=AXIS2_PLACEMENT_3D('',#4863,#3911,#3912);
#3443=AXIS2_PLACEMENT_3D('',#4866,#3915,#3916);
#3444=AXIS2_PLACEMENT_3D('',#4875,#3921,#3922);
#3445=AXIS2_PLACEMENT_3D('',#4881,#3926,#3927);
#3446=AXIS2_PLACEMENT_3D('',#4887,#3931,#3932);
#3447=AXIS2_PLACEMENT_3D('',#4890,#3935,#3936);
#3448=AXIS2_PLACEMENT_3D('',#4915,#3949,#3950);
#3449=AXIS2_PLACEMENT_3D('',#4940,#3963,#3964);
#3450=AXIS2_PLACEMENT_3D('',#4949,#3969,#3970);
#3451=AXIS2_PLACEMENT_3D('',#4950,#3971,#3972);
#3452=AXIS2_PLACEMENT_3D('',#4951,#3973,#3974);
#3453=AXIS2_PLACEMENT_3D('',#4952,#3975,#3976);
#3454=AXIS2_PLACEMENT_3D('',#4954,#3977,#3978);
#3455=AXIS2_PLACEMENT_3D('',#4957,#3980,#3981);
#3456=AXIS2_PLACEMENT_3D('',#4958,#3982,#3983);
#3457=AXIS2_PLACEMENT_3D('',#4964,#3987,#3988);
#3458=AXIS2_PLACEMENT_3D('',#4965,#3989,#3990);
#3459=AXIS2_PLACEMENT_3D('',#4966,#3991,#3992);
#3460=AXIS2_PLACEMENT_3D('',#4967,#3993,#3994);
#3461=AXIS2_PLACEMENT_3D('',#4968,#3995,#3996);
#3462=AXIS2_PLACEMENT_3D('',#4969,#3997,#3998);
#3463=AXIS2_PLACEMENT_3D('',#4970,#3999,#4000);
#3464=AXIS2_PLACEMENT_3D('',#4972,#4001,#4002);
#3465=AXIS2_PLACEMENT_3D('',#4974,#4003,#4004);
#3466=AXIS2_PLACEMENT_3D('',#4977,#4006,#4007);
#3467=AXIS2_PLACEMENT_3D('',#4979,#4008,#4009);
#3468=AXIS2_PLACEMENT_3D('',#4981,#4011,#4012);
#3469=AXIS2_PLACEMENT_3D('',#4983,#4013,#4014);
#3470=AXIS2_PLACEMENT_3D('',#4986,#4016,#4017);
#3471=AXIS2_PLACEMENT_3D('',#4988,#4018,#4019);
#3472=AXIS2_PLACEMENT_3D('',#4991,#4021,#4022);
#3473=AXIS2_PLACEMENT_3D('',#4992,#4023,#4024);
#3474=AXIS2_PLACEMENT_3D('',#4994,#4026,#4027);
#3475=AXIS2_PLACEMENT_3D('',#4996,#4029,#4030);
#3476=AXIS2_PLACEMENT_3D('',#4998,#4032,#4033);
#3477=AXIS2_PLACEMENT_3D('',#4999,#4034,#4035);
#3478=AXIS2_PLACEMENT_3D('',#5001,#4037,#4038);
#3479=AXIS2_PLACEMENT_3D('',#5002,#4039,#4040);
#3480=AXIS2_PLACEMENT_3D('',#5005,#4043,#4044);
#3481=AXIS2_PLACEMENT_3D('',#5007,#4046,#4047);
#3482=AXIS2_PLACEMENT_3D('',#5009,#4049,#4050);
#3483=AXIS2_PLACEMENT_3D('',#5010,#4051,#4052);
#3484=AXIS2_PLACEMENT_3D('',#5013,#4055,#4056);
#3485=AXIS2_PLACEMENT_3D('',#5015,#4058,#4059);
#3486=AXIS2_PLACEMENT_3D('',#5017,#4061,#4062);
#3487=AXIS2_PLACEMENT_3D('',#5018,#4063,#4064);
#3488=AXIS2_PLACEMENT_3D('',#5021,#4067,#4068);
#3489=AXIS2_PLACEMENT_3D('',#5023,#4070,#4071);
#3490=AXIS2_PLACEMENT_3D('',#5025,#4073,#4074);
#3491=AXIS2_PLACEMENT_3D('',#5026,#4075,#4076);
#3492=AXIS2_PLACEMENT_3D('',#5029,#4079,#4080);
#3493=AXIS2_PLACEMENT_3D('',#5031,#4082,#4083);
#3494=AXIS2_PLACEMENT_3D('',#5033,#4085,#4086);
#3865=DIRECTION('axis',(0.,0.,1.));
#3866=DIRECTION('refdir',(1.,0.,0.));
#3867=DIRECTION('center_axis',(-2.28847549044393E-17,-4.88654500275157E-16,
-1.));
#3868=DIRECTION('ref_axis',(0.,1.,-4.88654500275157E-16));
#3869=DIRECTION('',(-1.,-1.22464679914735E-16,2.28847549044394E-17));
#3870=DIRECTION('',(-1.22464679914735E-16,1.,-4.88654500275157E-16));
#3871=DIRECTION('',(-1.,-1.22464679914735E-16,2.28847549044394E-17));
#3872=DIRECTION('',(-1.22464679914735E-16,1.,-4.88654500275157E-16));
#3873=DIRECTION('',(-1.,1.32329071915688E-32,2.28847549044393E-17));
#3874=DIRECTION('',(-1.11827384717482E-32,1.,-4.88654500275157E-16));
#3875=DIRECTION('',(-1.,1.32329071915688E-32,2.28847549044393E-17));
#3876=DIRECTION('',(-1.11827384717482E-32,1.,-4.88654500275157E-16));
#3877=DIRECTION('',(1.,-1.32329071915688E-32,-2.28847549044393E-17));
#3878=DIRECTION('',(-1.11827384717482E-32,1.,-4.88654500275157E-16));
#3879=DIRECTION('',(1.,-1.32329071915688E-32,-2.28847549044393E-17));
#3880=DIRECTION('',(-1.11827384717482E-32,1.,-4.88654500275157E-16));
#3881=DIRECTION('center_axis',(2.28847549044393E-17,5.78241158658936E-16,
1.));
#3882=DIRECTION('ref_axis',(0.,-1.,5.78241158658936E-16));
#3883=DIRECTION('',(-1.,-1.22464679914735E-16,2.28847549044394E-17));
#3884=DIRECTION('',(-1.22464679914735E-16,1.,-5.78241158658936E-16));
#3885=DIRECTION('',(-1.,-1.22464679914735E-16,2.28847549044394E-17));
#3886=DIRECTION('',(-1.22464679914735E-16,1.,-5.78241158658936E-16));
#3887=DIRECTION('',(1.,-1.32329071915687E-32,-2.28847549044393E-17));
#3888=DIRECTION('',(1.32329071915687E-32,-1.,5.78241158658936E-16));
#3889=DIRECTION('',(1.,-1.32329071915687E-32,-2.28847549044393E-17));
#3890=DIRECTION('',(1.32329071915687E-32,-1.,5.78241158658936E-16));
#3891=DIRECTION('',(-1.,1.32329071915687E-32,2.28847549044393E-17));
#3892=DIRECTION('',(1.32329071915687E-32,-1.,5.78241158658936E-16));
#3893=DIRECTION('',(-1.,1.32329071915687E-32,2.28847549044393E-17));
#3894=DIRECTION('',(1.32329071915687E-32,-1.,5.78241158658936E-16));
#3895=DIRECTION('center_axis',(-1.710569414459E-48,-1.,5.78241158658936E-16));
#3896=DIRECTION('ref_axis',(1.82731431016009E-80,-5.78241158658936E-16,
-1.));
#3897=DIRECTION('',(2.28847549044393E-17,-5.78241158658936E-16,-1.));
#3898=DIRECTION('',(-1.,-1.32329071915688E-32,-2.28847549044394E-17));
#3899=DIRECTION('',(2.28847549044393E-17,-5.78241158658936E-16,-1.));
#3900=DIRECTION('',(1.,1.32329071915687E-32,2.28847549044393E-17));
#3901=DIRECTION('center_axis',(1.,1.710569414459E-48,2.28847549044393E-17));
#3902=DIRECTION('ref_axis',(-2.28847549044393E-17,0.,1.));
#3903=DIRECTION('',(1.64643319114981E-48,-1.,2.80257418429934E-33));
#3904=DIRECTION('',(2.28847549044393E-17,-5.78241158658936E-16,-1.));
#3905=DIRECTION('',(1.32329071915687E-32,1.,-5.78241158658936E-16));
#3906=DIRECTION('center_axis',(1.710569414459E-48,1.,-5.78241158658936E-16));
#3907=DIRECTION('ref_axis',(-1.82731431016009E-80,5.78241158658936E-16,
1.));
#3908=DIRECTION('',(1.,1.32329071915688E-32,2.28847549044394E-17));
#3909=DIRECTION('',(2.28847549044393E-17,-5.78241158658936E-16,-1.));
#3910=DIRECTION('',(-1.,-1.32329071915687E-32,-2.28847549044393E-17));
#3911=DIRECTION('center_axis',(-1.,-1.710569414459E-48,-2.28847549044393E-17));
#3912=DIRECTION('ref_axis',(2.28847549044393E-17,0.,-1.));
#3913=DIRECTION('',(-1.64643319114981E-48,1.,-2.80257418429934E-33));
#3914=DIRECTION('',(-1.32329071915687E-32,-1.,5.78241158658936E-16));
#3915=DIRECTION('center_axis',(-1.710569414459E-48,-1.,5.78241158658936E-16));
#3916=DIRECTION('ref_axis',(1.82731431016009E-80,-5.78241158658936E-16,
-1.));
#3917=DIRECTION('',(2.28847549044393E-17,-5.78241158658936E-16,-1.));
#3918=DIRECTION('',(-1.,-1.32329071915688E-32,-2.28847549044394E-17));
#3919=DIRECTION('',(2.28847549044393E-17,-5.78241158658936E-16,-1.));
#3920=DIRECTION('',(1.,1.32329071915687E-32,2.28847549044393E-17));
#3921=DIRECTION('center_axis',(-1.,-1.710569414459E-48,-2.28847549044393E-17));
#3922=DIRECTION('ref_axis',(2.28847549044393E-17,0.,-1.));
#3923=DIRECTION('',(-1.64643319114981E-48,1.,-2.80257418429934E-33));
#3924=DIRECTION('',(2.28847549044393E-17,-5.78241158658936E-16,-1.));
#3925=DIRECTION('',(-1.32329071915687E-32,-1.,5.78241158658936E-16));
#3926=DIRECTION('center_axis',(-1.710569414459E-48,-1.,5.78241158658936E-16));
#3927=DIRECTION('ref_axis',(1.82731431016009E-80,-5.78241158658936E-16,
-1.));
#3928=DIRECTION('',(-1.,-1.32329071915688E-32,-2.28847549044394E-17));
#3929=DIRECTION('',(2.28847549044393E-17,-5.78241158658936E-16,-1.));
#3930=DIRECTION('',(1.,1.32329071915687E-32,2.28847549044393E-17));
#3931=DIRECTION('center_axis',(-1.,-1.710569414459E-48,-2.28847549044393E-17));
#3932=DIRECTION('ref_axis',(2.28847549044393E-17,0.,-1.));
#3933=DIRECTION('',(-1.64643319114981E-48,1.,-2.80257418429934E-33));
#3934=DIRECTION('',(-1.32329071915687E-32,-1.,5.78241158658936E-16));
#3935=DIRECTION('center_axis',(2.28847549044394E-17,2.80257418429934E-33,
1.));
#3936=DIRECTION('ref_axis',(1.,4.56206030093224E-66,-2.28847549044394E-17));
#3937=DIRECTION('',(-1.,-1.22464679914735E-16,2.28847549044394E-17));
#3938=DIRECTION('',(-1.22464679914735E-16,1.,0.));
#3939=DIRECTION('',(-1.,-1.22464679914735E-16,2.28847549044394E-17));
#3940=DIRECTION('',(-1.22464679914735E-16,1.,0.));
#3941=DIRECTION('',(-1.,1.32329071915688E-32,2.28847549044394E-17));
#3942=DIRECTION('',(1.64643319114981E-48,1.,-2.80257418429934E-33));
#3943=DIRECTION('',(1.,-1.32329071915688E-32,-2.28847549044394E-17));
#3944=DIRECTION('',(-1.64643319114981E-48,-1.,2.80257418429934E-33));
#3945=DIRECTION('',(1.,-1.32329071915688E-32,-2.28847549044394E-17));
#3946=DIRECTION('',(1.64643319114981E-48,1.,-2.80257418429934E-33));
#3947=DIRECTION('',(1.,-1.32329071915688E-32,-2.28847549044394E-17));
#3948=DIRECTION('',(1.64643319114981E-48,1.,-2.80257418429934E-33));
#3949=DIRECTION('center_axis',(-2.28847549044393E-17,-5.78241158658936E-16,
-1.));
#3950=DIRECTION('ref_axis',(0.,1.,-5.78241158658936E-16));
#3951=DIRECTION('',(-1.,-1.22464679914735E-16,2.28847549044394E-17));
#3952=DIRECTION('',(-1.22464679914735E-16,1.,-5.78241158658936E-16));
#3953=DIRECTION('',(-1.,-1.22464679914735E-16,2.28847549044394E-17));
#3954=DIRECTION('',(-1.22464679914735E-16,1.,-5.78241158658936E-16));
#3955=DIRECTION('',(-1.,1.32329071915687E-32,2.28847549044393E-17));
#3956=DIRECTION('',(1.32329071915687E-32,-1.,5.78241158658936E-16));
#3957=DIRECTION('',(1.,-1.32329071915687E-32,-2.28847549044393E-17));
#3958=DIRECTION('',(-1.32329071915687E-32,1.,-5.78241158658936E-16));
#3959=DIRECTION('',(-1.,1.32329071915687E-32,2.28847549044393E-17));
#3960=DIRECTION('',(1.32329071915687E-32,-1.,5.78241158658936E-16));
#3961=DIRECTION('',(-1.,1.32329071915687E-32,2.28847549044393E-17));
#3962=DIRECTION('',(1.32329071915687E-32,-1.,5.78241158658936E-16));
#3963=DIRECTION('center_axis',(1.22464679914735E-16,-1.,5.78241158658936E-16));
#3964=DIRECTION('ref_axis',(1.41228329145101E-48,-5.78241158658936E-16,
-1.));
#3965=DIRECTION('',(2.28847549044393E-17,5.78241158658936E-16,1.));
#3966=DIRECTION('',(-1.,-1.22464679914735E-16,2.28847549044394E-17));
#3967=DIRECTION('',(2.28847549044393E-17,5.78241158658936E-16,1.));
#3968=DIRECTION('',(-1.,-1.22464679914735E-16,2.28847549044394E-17));
#3969=DIRECTION('center_axis',(-1.,-1.22464679914735E-16,2.28847549044394E-17));
#3970=DIRECTION('ref_axis',(1.22464679914735E-16,-1.,-1.1877739243467E-49));
#3971=DIRECTION('center_axis',(-1.,-1.22464679914735E-16,2.28847549044394E-17));
#3972=DIRECTION('ref_axis',(-2.28847549044394E-17,-2.80257418429934E-33,
-1.));
#3973=DIRECTION('center_axis',(-1.,-1.22464679914735E-16,2.28847549044394E-17));
#3974=DIRECTION('ref_axis',(-2.28847549044394E-17,-2.80257418429934E-33,
-1.));
#3975=DIRECTION('center_axis',(-1.,-1.22464679914735E-16,2.28847549044394E-17));
#3976=DIRECTION('ref_axis',(1.22464679914735E-16,-1.,-1.1877739243467E-49));
#3977=DIRECTION('center_axis',(-1.,-1.22464679914735E-16,2.28847549044394E-17));
#3978=DIRECTION('ref_axis',(-2.28847549044394E-17,-2.80257418429934E-33,
-1.));
#3979=DIRECTION('',(-1.,-1.22464679914735E-16,2.28847549044394E-17));
#3980=DIRECTION('center_axis',(-1.,-1.22464679914735E-16,2.28847549044394E-17));
#3981=DIRECTION('ref_axis',(-2.28847549044394E-17,-2.80257418429934E-33,
-1.));
#3982=DIRECTION('center_axis',(-1.22464679914735E-16,1.,-5.78241158658936E-16));
#3983=DIRECTION('ref_axis',(-1.41228329145101E-48,5.78241158658936E-16,
1.));
#3984=DIRECTION('',(2.28847549044393E-17,5.78241158658936E-16,1.));
#3985=DIRECTION('',(-1.,-1.22464679914735E-16,2.28847549044394E-17));
#3986=DIRECTION('',(2.28847549044393E-17,5.78241158658936E-16,1.));
#3987=DIRECTION('center_axis',(-1.,-1.22464679914735E-16,2.28847549044394E-17));
#3988=DIRECTION('ref_axis',(1.22464679914735E-16,-1.,-1.1877739243467E-49));
#3989=DIRECTION('center_axis',(-1.,-1.22464679914735E-16,2.28847549044394E-17));
#3990=DIRECTION('ref_axis',(-2.28847549044394E-17,-2.80257418429934E-33,
-1.));
#3991=DIRECTION('center_axis',(-1.,-1.22464679914735E-16,2.28847549044394E-17));
#3992=DIRECTION('ref_axis',(-2.28847549044394E-17,-2.80257418429934E-33,
-1.));
#3993=DIRECTION('center_axis',(-1.,-1.22464679914735E-16,2.28847549044394E-17));
#3994=DIRECTION('ref_axis',(1.22464679914735E-16,-1.,-1.1877739243467E-49));
#3995=DIRECTION('center_axis',(-1.,-1.22464679914735E-16,2.28847549044394E-17));
#3996=DIRECTION('ref_axis',(-2.28847549044394E-17,-2.80257418429934E-33,
-1.));
#3997=DIRECTION('center_axis',(-1.,-1.22464679914735E-16,2.28847549044394E-17));
#3998=DIRECTION('ref_axis',(-2.28847549044394E-17,-2.80257418429934E-33,
-1.));
#3999=DIRECTION('center_axis',(-1.,-1.22464679914735E-16,2.28847549044394E-17));
#4000=DIRECTION('ref_axis',(1.22464679914735E-16,-1.,-1.1877739243467E-49));
#4001=DIRECTION('center_axis',(-1.,-1.22464679914735E-16,2.28847549044394E-17));
#4002=DIRECTION('ref_axis',(-2.28847549044394E-17,-2.80257418429934E-33,
-1.));
#4003=DIRECTION('center_axis',(-1.,-1.22464679914735E-16,2.28847549044394E-17));
#4004=DIRECTION('ref_axis',(-2.28847549044394E-17,-2.80257418429934E-33,
-1.));
#4005=DIRECTION('',(2.28847549044393E-17,4.88654500275157E-16,1.));
#4006=DIRECTION('center_axis',(-1.,-1.22464679914735E-16,2.28847549044394E-17));
#4007=DIRECTION('ref_axis',(-2.28847549044394E-17,-2.80257418429934E-33,
-1.));
#4008=DIRECTION('center_axis',(-1.,-1.22464679914735E-16,2.28847549044394E-17));
#4009=DIRECTION('ref_axis',(-2.28847549044394E-17,-2.80257418429934E-33,
-1.));
#4010=DIRECTION('',(2.28847549044393E-17,4.88654500275157E-16,1.));
#4011=DIRECTION('center_axis',(-1.,-1.22464679914735E-16,2.28847549044394E-17));
#4012=DIRECTION('ref_axis',(1.22464679914735E-16,-1.,-1.1877739243467E-49));
#4013=DIRECTION('center_axis',(-1.,-1.22464679914735E-16,2.28847549044394E-17));
#4014=DIRECTION('ref_axis',(-2.28847549044394E-17,-2.80257418429934E-33,
-1.));
#4015=DIRECTION('',(2.28847549044393E-17,4.88654500275157E-16,1.));
#4016=DIRECTION('center_axis',(-1.,-1.22464679914735E-16,2.28847549044394E-17));
#4017=DIRECTION('ref_axis',(-2.28847549044394E-17,-2.80257418429934E-33,
-1.));
#4018=DIRECTION('center_axis',(-1.,-1.22464679914735E-16,2.28847549044394E-17));
#4019=DIRECTION('ref_axis',(-2.28847549044394E-17,-2.80257418429934E-33,
-1.));
#4020=DIRECTION('',(2.28847549044393E-17,4.88654500275157E-16,1.));
#4021=DIRECTION('center_axis',(-1.,-1.22464679914735E-16,2.28847549044394E-17));
#4022=DIRECTION('ref_axis',(-2.28847549044394E-17,-2.80257418429934E-33,
-1.));
#4023=DIRECTION('center_axis',(-1.,-1.22464679914735E-16,2.28847549044394E-17));
#4024=DIRECTION('ref_axis',(1.22464679914735E-16,-1.,-1.1877739243467E-49));
#4025=DIRECTION('',(-1.,-1.22464679914735E-16,2.28847549044394E-17));
#4026=DIRECTION('center_axis',(-1.,-1.22464679914735E-16,2.28847549044394E-17));
#4027=DIRECTION('ref_axis',(1.22464679914735E-16,-1.,-1.1877739243467E-49));
#4028=DIRECTION('',(-1.,-1.22464679914735E-16,2.28847549044394E-17));
#4029=DIRECTION('center_axis',(-1.22464679914735E-16,1.,-4.88654500275157E-16));
#4030=DIRECTION('ref_axis',(-3.23663765428249E-48,4.88654500275157E-16,
1.));
#4031=DIRECTION('',(-1.,-1.22464679914735E-16,2.28847549044394E-17));
#4032=DIRECTION('center_axis',(-1.,-1.22464679914735E-16,2.28847549044394E-17));
#4033=DIRECTION('ref_axis',(1.22464679914735E-16,-1.,-1.1877739243467E-49));
#4034=DIRECTION('center_axis',(-1.,-1.22464679914735E-16,2.28847549044394E-17));
#4035=DIRECTION('ref_axis',(1.22464679914735E-16,-1.,-1.1877739243467E-49));
#4036=DIRECTION('',(-1.,-1.22464679914735E-16,2.28847549044394E-17));
#4037=DIRECTION('center_axis',(1.22464679914735E-16,-1.,4.88654500275157E-16));
#4038=DIRECTION('ref_axis',(3.23663765428249E-48,-4.88654500275157E-16,
-1.));
#4039=DIRECTION('center_axis',(1.,-1.710569414459E-48,-2.28847549044393E-17));
#4040=DIRECTION('ref_axis',(-2.28847549044393E-17,0.,-1.));
#4041=DIRECTION('',(-2.28847549044393E-17,-5.78241158658936E-16,-1.));
#4042=DIRECTION('',(-2.28847549044393E-17,-5.78241158658936E-16,-1.));
#4043=DIRECTION('center_axis',(1.710569414459E-48,-1.,5.78241158658936E-16));
#4044=DIRECTION('ref_axis',(-1.82731431016009E-80,-5.78241158658936E-16,
-1.));
#4045=DIRECTION('',(-2.28847549044393E-17,-5.78241158658936E-16,-1.));
#4046=DIRECTION('center_axis',(-1.,1.710569414459E-48,2.28847549044393E-17));
#4047=DIRECTION('ref_axis',(2.28847549044393E-17,0.,1.));
#4048=DIRECTION('',(-2.28847549044393E-17,-5.78241158658936E-16,-1.));
#4049=DIRECTION('center_axis',(-1.710569414459E-48,1.,-5.78241158658936E-16));
#4050=DIRECTION('ref_axis',(1.82731431016009E-80,5.78241158658936E-16,1.));
#4051=DIRECTION('center_axis',(1.,-1.710569414459E-48,-2.28847549044393E-17));
#4052=DIRECTION('ref_axis',(-2.28847549044393E-17,0.,-1.));
#4053=DIRECTION('',(-2.28847549044393E-17,-5.78241158658936E-16,-1.));
#4054=DIRECTION('',(-2.28847549044393E-17,-5.78241158658936E-16,-1.));
#4055=DIRECTION('center_axis',(1.710569414459E-48,-1.,5.78241158658936E-16));
#4056=DIRECTION('ref_axis',(-1.82731431016009E-80,-5.78241158658936E-16,
-1.));
#4057=DIRECTION('',(-2.28847549044393E-17,-5.78241158658936E-16,-1.));
#4058=DIRECTION('center_axis',(1.,-1.710569414459E-48,-2.28847549044393E-17));
#4059=DIRECTION('ref_axis',(-2.28847549044393E-17,0.,-1.));
#4060=DIRECTION('',(-2.28847549044393E-17,-5.78241158658936E-16,-1.));
#4061=DIRECTION('center_axis',(1.710569414459E-48,-1.,5.78241158658936E-16));
#4062=DIRECTION('ref_axis',(-1.82731431016009E-80,-5.78241158658936E-16,
-1.));
#4063=DIRECTION('center_axis',(-1.,1.710569414459E-48,2.28847549044393E-17));
#4064=DIRECTION('ref_axis',(2.28847549044393E-17,0.,1.));
#4065=DIRECTION('',(2.28847549044393E-17,5.78241158658936E-16,1.));
#4066=DIRECTION('',(2.28847549044393E-17,5.78241158658936E-16,1.));
#4067=DIRECTION('center_axis',(1.710569414459E-48,-1.,5.78241158658936E-16));
#4068=DIRECTION('ref_axis',(-1.82731431016009E-80,-5.78241158658936E-16,
-1.));
#4069=DIRECTION('',(2.28847549044393E-17,5.78241158658936E-16,1.));
#4070=DIRECTION('center_axis',(-1.,1.710569414459E-48,2.28847549044393E-17));
#4071=DIRECTION('ref_axis',(2.28847549044393E-17,0.,1.));
#4072=DIRECTION('',(2.28847549044393E-17,5.78241158658936E-16,1.));
#4073=DIRECTION('center_axis',(1.710569414459E-48,-1.,5.78241158658936E-16));
#4074=DIRECTION('ref_axis',(-1.82731431016009E-80,-5.78241158658936E-16,
-1.));
#4075=DIRECTION('center_axis',(-1.,1.710569414459E-48,2.28847549044393E-17));
#4076=DIRECTION('ref_axis',(2.28847549044393E-17,0.,1.));
#4077=DIRECTION('',(2.28847549044393E-17,5.78241158658936E-16,1.));
#4078=DIRECTION('',(2.28847549044393E-17,5.78241158658936E-16,1.));
#4079=DIRECTION('center_axis',(-1.710569414459E-48,1.,-5.78241158658936E-16));
#4080=DIRECTION('ref_axis',(1.82731431016009E-80,5.78241158658936E-16,1.));
#4081=DIRECTION('',(2.28847549044393E-17,5.78241158658936E-16,1.));
#4082=DIRECTION('center_axis',(-1.,1.710569414459E-48,2.28847549044393E-17));
#4083=DIRECTION('ref_axis',(2.28847549044393E-17,0.,1.));
#4084=DIRECTION('',(2.28847549044393E-17,5.78241158658936E-16,1.));
#4085=DIRECTION('center_axis',(-1.710569414459E-48,1.,-5.78241158658936E-16));
#4086=DIRECTION('ref_axis',(1.82731431016009E-80,5.78241158658936E-16,1.));
#4791=CARTESIAN_POINT('',(0.,0.,0.));
#4792=CARTESIAN_POINT('Origin',(550.,850.,2188.));
#4793=CARTESIAN_POINT('',(550.,835.8,2188.));
#4794=CARTESIAN_POINT('',(-550.,835.8,2188.));
#4795=CARTESIAN_POINT('',(550.,835.8,2188.));
#4796=CARTESIAN_POINT('',(-550.,864.2,2188.));
#4797=CARTESIAN_POINT('',(-550.,850.,2188.));
#4798=CARTESIAN_POINT('',(550.,864.2,2188.));
#4799=CARTESIAN_POINT('',(550.,864.2,2188.));
#4800=CARTESIAN_POINT('',(550.,850.,2188.));
#4801=CARTESIAN_POINT('',(290.,840.,2188.));
#4802=CARTESIAN_POINT('',(280.,840.,2188.));
#4803=CARTESIAN_POINT('',(550.,840.,2188.));
#4804=CARTESIAN_POINT('',(290.,860.,2188.));
#4805=CARTESIAN_POINT('',(290.,850.,2188.));
#4806=CARTESIAN_POINT('',(280.,860.,2188.));
#4807=CARTESIAN_POINT('',(550.,860.,2188.));
#4808=CARTESIAN_POINT('',(280.,850.,2188.));
#4809=CARTESIAN_POINT('',(-290.,840.,2188.));
#4810=CARTESIAN_POINT('',(-280.,840.,2188.));
#4811=CARTESIAN_POINT('',(550.,840.,2188.));
#4812=CARTESIAN_POINT('',(-280.,860.,2188.));
#4813=CARTESIAN_POINT('',(-280.,850.,2188.));
#4814=CARTESIAN_POINT('',(-290.,860.,2188.));
#4815=CARTESIAN_POINT('',(550.,860.,2188.));
#4816=CARTESIAN_POINT('',(-290.,850.,2188.));
#4817=CARTESIAN_POINT('Origin',(550.,850.,2192.));
#4818=CARTESIAN_POINT('',(550.,868.,2192.));
#4819=CARTESIAN_POINT('',(-550.,868.,2192.));
#4820=CARTESIAN_POINT('',(550.,868.,2192.));
#4821=CARTESIAN_POINT('',(-550.,832.,2192.));
#4822=CARTESIAN_POINT('',(-550.,850.,2192.));
#4823=CARTESIAN_POINT('',(550.,832.,2192.));
#4824=CARTESIAN_POINT('',(550.,832.,2192.));
#4825=CARTESIAN_POINT('',(550.,850.,2192.));
#4826=CARTESIAN_POINT('',(280.,860.,2192.));
#4827=CARTESIAN_POINT('',(290.,860.,2192.));
#4828=CARTESIAN_POINT('',(285.,860.,2192.));
#4829=CARTESIAN_POINT('',(290.,840.,2192.));
#4830=CARTESIAN_POINT('',(290.,850.,2192.));
#4831=CARTESIAN_POINT('',(280.,840.,2192.));
#4832=CARTESIAN_POINT('',(285.,840.,2192.));
#4833=CARTESIAN_POINT('',(280.,850.,2192.));
#4834=CARTESIAN_POINT('',(-280.,860.,2192.));
#4835=CARTESIAN_POINT('',(-290.,860.,2192.));
#4836=CARTESIAN_POINT('',(-285.,860.,2192.));
#4837=CARTESIAN_POINT('',(-280.,840.,2192.));
#4838=CARTESIAN_POINT('',(-280.,850.,2192.));
#4839=CARTESIAN_POINT('',(-290.,840.,2192.));
#4840=CARTESIAN_POINT('',(-285.,840.,2192.));
#4841=CARTESIAN_POINT('',(-290.,850.,2192.));
#4842=CARTESIAN_POINT('Origin',(378.,856.,2177.));
#4843=CARTESIAN_POINT('',(381.,856.,2156.));
#4844=CARTESIAN_POINT('',(381.,856.,2152.));
#4845=CARTESIAN_POINT('',(381.,856.,2177.));
#4846=CARTESIAN_POINT('',(375.,856.,2156.));
#4847=CARTESIAN_POINT('',(-550.,856.,2156.));
#4848=CARTESIAN_POINT('',(375.,856.,2152.));
#4849=CARTESIAN_POINT('',(375.,856.,2177.));
#4850=CARTESIAN_POINT('',(378.,856.,2152.));
#4851=CARTESIAN_POINT('Origin',(375.,850.,2177.));
#4852=CARTESIAN_POINT('',(375.,844.,2156.));
#4853=CARTESIAN_POINT('',(375.,850.,2156.));
#4854=CARTESIAN_POINT('',(375.,844.,2152.));
#4855=CARTESIAN_POINT('',(375.,844.,2177.));
#4856=CARTESIAN_POINT('',(375.,850.,2152.));
#4857=CARTESIAN_POINT('Origin',(378.,844.,2177.));
#4858=CARTESIAN_POINT('',(381.,844.,2156.));
#4859=CARTESIAN_POINT('',(-550.,844.,2156.));
#4860=CARTESIAN_POINT('',(381.,844.,2152.));
#4861=CARTESIAN_POINT('',(381.,844.,2177.));
#4862=CARTESIAN_POINT('',(378.,844.,2152.));
#4863=CARTESIAN_POINT('Origin',(381.,850.,2177.));
#4864=CARTESIAN_POINT('',(381.,850.,2156.));
#4865=CARTESIAN_POINT('',(381.,850.,2152.));
#4866=CARTESIAN_POINT('Origin',(342.,856.,2177.));
#4867=CARTESIAN_POINT('',(345.,856.,2156.));
#4868=CARTESIAN_POINT('',(345.,856.,2152.));
#4869=CARTESIAN_POINT('',(345.,856.,2177.));
#4870=CARTESIAN_POINT('',(339.,856.,2156.));
#4871=CARTESIAN_POINT('',(-550.,856.,2156.));
#4872=CARTESIAN_POINT('',(339.,856.,2152.));
#4873=CARTESIAN_POINT('',(339.,856.,2177.));
#4874=CARTESIAN_POINT('',(342.,856.,2152.));
#4875=CARTESIAN_POINT('Origin',(339.,850.,2177.));
#4876=CARTESIAN_POINT('',(339.,844.,2156.));
#4877=CARTESIAN_POINT('',(339.,850.,2156.));
#4878=CARTESIAN_POINT('',(339.,844.,2152.));
#4879=CARTESIAN_POINT('',(339.,844.,2177.));
#4880=CARTESIAN_POINT('',(339.,850.,2152.));
#4881=CARTESIAN_POINT('Origin',(342.,844.,2177.));
#4882=CARTESIAN_POINT('',(345.,844.,2156.));
#4883=CARTESIAN_POINT('',(-550.,844.,2156.));
#4884=CARTESIAN_POINT('',(345.,844.,2152.));
#4885=CARTESIAN_POINT('',(345.,844.,2177.));
#4886=CARTESIAN_POINT('',(342.,844.,2152.));
#4887=CARTESIAN_POINT('Origin',(345.,850.,2177.));
#4888=CARTESIAN_POINT('',(345.,850.,2156.));
#4889=CARTESIAN_POINT('',(345.,850.,2152.));
#4890=CARTESIAN_POINT('Origin',(550.,850.,2156.));
#4891=CARTESIAN_POINT('',(550.,864.2,2156.));
#4892=CARTESIAN_POINT('',(-550.,864.2,2156.));
#4893=CARTESIAN_POINT('',(550.,864.2,2156.));
#4894=CARTESIAN_POINT('',(-550.,835.8,2156.));
#4895=CARTESIAN_POINT('',(-550.,850.,2156.));
#4896=CARTESIAN_POINT('',(550.,835.8,2156.));
#4897=CARTESIAN_POINT('',(550.,835.8,2156.));
#4898=CARTESIAN_POINT('',(550.,850.,2156.));
#4899=CARTESIAN_POINT('',(-375.,844.,2156.));
#4900=CARTESIAN_POINT('',(-381.,844.,2156.));
#4901=CARTESIAN_POINT('',(550.,844.,2156.));
#4902=CARTESIAN_POINT('',(-381.,856.,2156.));
#4903=CARTESIAN_POINT('',(-381.,850.,2156.));
#4904=CARTESIAN_POINT('',(-375.,856.,2156.));
#4905=CARTESIAN_POINT('',(550.,856.,2156.));
#4906=CARTESIAN_POINT('',(-375.,850.,2156.));
#4907=CARTESIAN_POINT('',(-345.,844.,2156.));
#4908=CARTESIAN_POINT('',(-339.,844.,2156.));
#4909=CARTESIAN_POINT('',(550.,844.,2156.));
#4910=CARTESIAN_POINT('',(-345.,856.,2156.));
#4911=CARTESIAN_POINT('',(-345.,850.,2156.));
#4912=CARTESIAN_POINT('',(-339.,856.,2156.));
#4913=CARTESIAN_POINT('',(550.,856.,2156.));
#4914=CARTESIAN_POINT('',(-339.,850.,2156.));
#4915=CARTESIAN_POINT('Origin',(550.,850.,2152.));
#4916=CARTESIAN_POINT('',(550.,832.,2152.));
#4917=CARTESIAN_POINT('',(-550.,832.,2152.));
#4918=CARTESIAN_POINT('',(550.,832.,2152.));
#4919=CARTESIAN_POINT('',(-550.,868.,2152.));
#4920=CARTESIAN_POINT('',(-550.,850.,2152.));
#4921=CARTESIAN_POINT('',(550.,868.,2152.));
#4922=CARTESIAN_POINT('',(550.,868.,2152.));
#4923=CARTESIAN_POINT('',(550.,850.,2152.));
#4924=CARTESIAN_POINT('',(-375.,856.,2152.));
#4925=CARTESIAN_POINT('',(-381.,856.,2152.));
#4926=CARTESIAN_POINT('',(-378.,856.,2152.));
#4927=CARTESIAN_POINT('',(-381.,844.,2152.));
#4928=CARTESIAN_POINT('',(-381.,850.,2152.));
#4929=CARTESIAN_POINT('',(-375.,844.,2152.));
#4930=CARTESIAN_POINT('',(-378.,844.,2152.));
#4931=CARTESIAN_POINT('',(-375.,850.,2152.));
#4932=CARTESIAN_POINT('',(-339.,856.,2152.));
#4933=CARTESIAN_POINT('',(-345.,856.,2152.));
#4934=CARTESIAN_POINT('',(-342.,856.,2152.));
#4935=CARTESIAN_POINT('',(-345.,844.,2152.));
#4936=CARTESIAN_POINT('',(-345.,850.,2152.));
#4937=CARTESIAN_POINT('',(-339.,844.,2152.));
#4938=CARTESIAN_POINT('',(-342.,844.,2152.));
#4939=CARTESIAN_POINT('',(-339.,850.,2152.));
#4940=CARTESIAN_POINT('Origin',(550.,830.,2172.));
#4941=CARTESIAN_POINT('',(-550.,830.,2154.));
#4942=CARTESIAN_POINT('',(-550.,830.,2190.));
#4943=CARTESIAN_POINT('',(-550.,830.,2172.));
#4944=CARTESIAN_POINT('',(550.,830.,2154.));
#4945=CARTESIAN_POINT('',(550.,830.,2154.));
#4946=CARTESIAN_POINT('',(550.,830.,2190.));
#4947=CARTESIAN_POINT('',(550.,830.,2172.));
#4948=CARTESIAN_POINT('',(550.,830.,2190.));
#4949=CARTESIAN_POINT('Origin',(550.,832.,2154.));
#4950=CARTESIAN_POINT('Origin',(-550.,832.,2154.));
#4951=CARTESIAN_POINT('Origin',(550.,832.,2154.));
#4952=CARTESIAN_POINT('Origin',(550.,868.,2154.));
#4953=CARTESIAN_POINT('',(-550.,870.,2154.));
#4954=CARTESIAN_POINT('Origin',(-550.,868.,2154.));
#4955=CARTESIAN_POINT('',(550.,870.,2154.));
#4956=CARTESIAN_POINT('',(550.,870.,2154.));
#4957=CARTESIAN_POINT('Origin',(550.,868.,2154.));
#4958=CARTESIAN_POINT('Origin',(550.,870.,2172.));
#4959=CARTESIAN_POINT('',(-550.,870.,2190.));
#4960=CARTESIAN_POINT('',(-550.,870.,2172.));
#4961=CARTESIAN_POINT('',(550.,870.,2190.));
#4962=CARTESIAN_POINT('',(550.,870.,2190.));
#4963=CARTESIAN_POINT('',(550.,870.,2172.));
#4964=CARTESIAN_POINT('Origin',(550.,868.,2190.));
#4965=CARTESIAN_POINT('Origin',(-550.,868.,2190.));
#4966=CARTESIAN_POINT('Origin',(550.,868.,2190.));
#4967=CARTESIAN_POINT('Origin',(550.,832.,2190.));
#4968=CARTESIAN_POINT('Origin',(-550.,832.,2190.));
#4969=CARTESIAN_POINT('Origin',(550.,832.,2190.));
#4970=CARTESIAN_POINT('Origin',(-550.,850.,2172.));
#4971=CARTESIAN_POINT('',(-550.,866.,2186.2));
#4972=CARTESIAN_POINT('Origin',(-550.,864.2,2186.2));
#4973=CARTESIAN_POINT('',(-550.,834.,2186.2));
#4974=CARTESIAN_POINT('Origin',(-550.,835.8,2186.2));
#4975=CARTESIAN_POINT('',(-550.,834.,2157.8));
#4976=CARTESIAN_POINT('',(-550.,834.,2172.));
#4977=CARTESIAN_POINT('Origin',(-550.,835.8,2157.8));
#4978=CARTESIAN_POINT('',(-550.,866.,2157.8));
#4979=CARTESIAN_POINT('Origin',(-550.,864.2,2157.8));
#4980=CARTESIAN_POINT('',(-550.,866.,2172.));
#4981=CARTESIAN_POINT('Origin',(550.,850.,2172.));
#4982=CARTESIAN_POINT('',(550.,866.,2186.2));
#4983=CARTESIAN_POINT('Origin',(550.,864.2,2186.2));
#4984=CARTESIAN_POINT('',(550.,866.,2157.8));
#4985=CARTESIAN_POINT('',(550.,866.,2172.));
#4986=CARTESIAN_POINT('Origin',(550.,864.2,2157.8));
#4987=CARTESIAN_POINT('',(550.,834.,2157.8));
#4988=CARTESIAN_POINT('Origin',(550.,835.8,2157.8));
#4989=CARTESIAN_POINT('',(550.,834.,2186.2));
#4990=CARTESIAN_POINT('',(550.,834.,2172.));
#4991=CARTESIAN_POINT('Origin',(550.,835.8,2186.2));
#4992=CARTESIAN_POINT('Origin',(550.,864.2,2157.8));
#4993=CARTESIAN_POINT('',(550.,866.,2157.8));
#4994=CARTESIAN_POINT('Origin',(550.,835.8,2157.8));
#4995=CARTESIAN_POINT('',(550.,834.,2157.8));
#4996=CARTESIAN_POINT('Origin',(550.,834.,2172.));
#4997=CARTESIAN_POINT('',(550.,834.,2186.2));
#4998=CARTESIAN_POINT('Origin',(550.,835.8,2186.2));
#4999=CARTESIAN_POINT('Origin',(550.,864.2,2186.2));
#5000=CARTESIAN_POINT('',(550.,866.,2186.2));
#5001=CARTESIAN_POINT('Origin',(550.,866.,2172.));
#5002=CARTESIAN_POINT('Origin',(-381.,850.,2177.));
#5003=CARTESIAN_POINT('',(-381.,844.,2177.));
#5004=CARTESIAN_POINT('',(-381.,856.,2177.));
#5005=CARTESIAN_POINT('Origin',(-378.,856.,2177.));
#5006=CARTESIAN_POINT('',(-375.,856.,2177.));
#5007=CARTESIAN_POINT('Origin',(-375.,850.,2177.));
#5008=CARTESIAN_POINT('',(-375.,844.,2177.));
#5009=CARTESIAN_POINT('Origin',(-378.,844.,2177.));
#5010=CARTESIAN_POINT('Origin',(-345.,850.,2177.));
#5011=CARTESIAN_POINT('',(-345.,844.,2177.));
#5012=CARTESIAN_POINT('',(-345.,856.,2177.));
#5013=CARTESIAN_POINT('Origin',(-342.,856.,2177.));
#5014=CARTESIAN_POINT('',(-339.,856.,2177.));
#5015=CARTESIAN_POINT('Origin',(-339.,850.,2177.));
#5016=CARTESIAN_POINT('',(-339.,844.,2177.));
#5017=CARTESIAN_POINT('Origin',(-342.,844.,2177.));
#5018=CARTESIAN_POINT('Origin',(290.,850.,2167.));
#5019=CARTESIAN_POINT('',(290.,840.,2167.));
#5020=CARTESIAN_POINT('',(290.,860.,2167.));
#5021=CARTESIAN_POINT('Origin',(285.,860.,2167.));
#5022=CARTESIAN_POINT('',(280.,860.,2167.));
#5023=CARTESIAN_POINT('Origin',(280.,850.,2167.));
#5024=CARTESIAN_POINT('',(280.,840.,2167.));
#5025=CARTESIAN_POINT('Origin',(285.,840.,2167.));
#5026=CARTESIAN_POINT('Origin',(-280.,850.,2167.));
#5027=CARTESIAN_POINT('',(-280.,840.,2167.));
#5028=CARTESIAN_POINT('',(-280.,860.,2167.));
#5029=CARTESIAN_POINT('Origin',(-285.,860.,2167.));
#5030=CARTESIAN_POINT('',(-290.,860.,2167.));
#5031=CARTESIAN_POINT('Origin',(-290.,850.,2167.));
#5032=CARTESIAN_POINT('',(-290.,840.,2167.));
#5033=CARTESIAN_POINT('Origin',(-285.,840.,2167.));
#5490=UNCERTAINTY_MEASURE_WITH_UNIT(LENGTH_MEASURE(0.01),#5506,
'DISTANCE_ACCURACY_VALUE',
'Maximum model space distance between geometric entities at asserted c
onnectivities');
#5496=UNCERTAINTY_MEASURE_WITH_UNIT(LENGTH_MEASURE(0.01),#5506,
'DISTANCE_ACCURACY_VALUE',
'Maximum model space distance between geometric entities at asserted c
onnectivities');
#5499=(
GEOMETRIC_REPRESENTATION_CONTEXT(3)
GLOBAL_UNCERTAINTY_ASSIGNED_CONTEXT((#5490))
GLOBAL_UNIT_ASSIGNED_CONTEXT((#5506,#5508,#5509))
REPRESENTATION_CONTEXT('','3D')
);
#5505=(
GEOMETRIC_REPRESENTATION_CONTEXT(3)
GLOBAL_UNCERTAINTY_ASSIGNED_CONTEXT((#5496))
GLOBAL_UNIT_ASSIGNED_CONTEXT((#5506,#5508,#5509))
REPRESENTATION_CONTEXT('','3D')
);
#5506=(
LENGTH_UNIT()
NAMED_UNIT(*)
SI_UNIT(.MILLI.,.METRE.)
);
#5508=(
NAMED_UNIT(*)
PLANE_ANGLE_UNIT()
SI_UNIT($,.RADIAN.)
);
#5509=(
NAMED_UNIT(*)
SI_UNIT($,.STERADIAN.)
SOLID_ANGLE_UNIT()
);
#5512=SHAPE_DEFINITION_REPRESENTATION(#5520,#5538);
#5520=PRODUCT_DEFINITION_SHAPE('',$,#5547);
#5538=SHAPE_REPRESENTATION('',(#3436),#5499);
#5544=PRODUCT_DEFINITION_CONTEXT('part definition',#5570,'design');
#5547=PRODUCT_DEFINITION('Mast-top-hinge','Mast-top-hinge',#5555,#5544);
#5555=PRODUCT_DEFINITION_FORMATION('',$,#5574);
#5570=APPLICATION_CONTEXT(
'Core Data for Automotive Mechanical Design Process');
#5571=PRODUCT_CONTEXT('part definition',#5570,'mechanical');
#5574=PRODUCT('Mast-top-hinge','Mast-top-hinge',
'40x40x3mm-2pcs-third-mast-top-hinge',(#5571));
#5582=PRESENTATION_STYLE_ASSIGNMENT((#5590));
#5590=SURFACE_STYLE_USAGE(.BOTH.,#5598);
#5598=SURFACE_SIDE_STYLE('',(#5606));
#5606=SURFACE_STYLE_FILL_AREA(#5614);
#5614=FILL_AREA_STYLE('Opaque(196,226,243)',(#5622));
#5622=FILL_AREA_STYLE_COLOUR('Opaque(196,226,243)',#5630);
#5630=COLOUR_RGB('Opaque(196,226,243)', 0.66274510, 0.83137255, 0.94901961);
ENDSEC;
END-ISO-10303-21;
